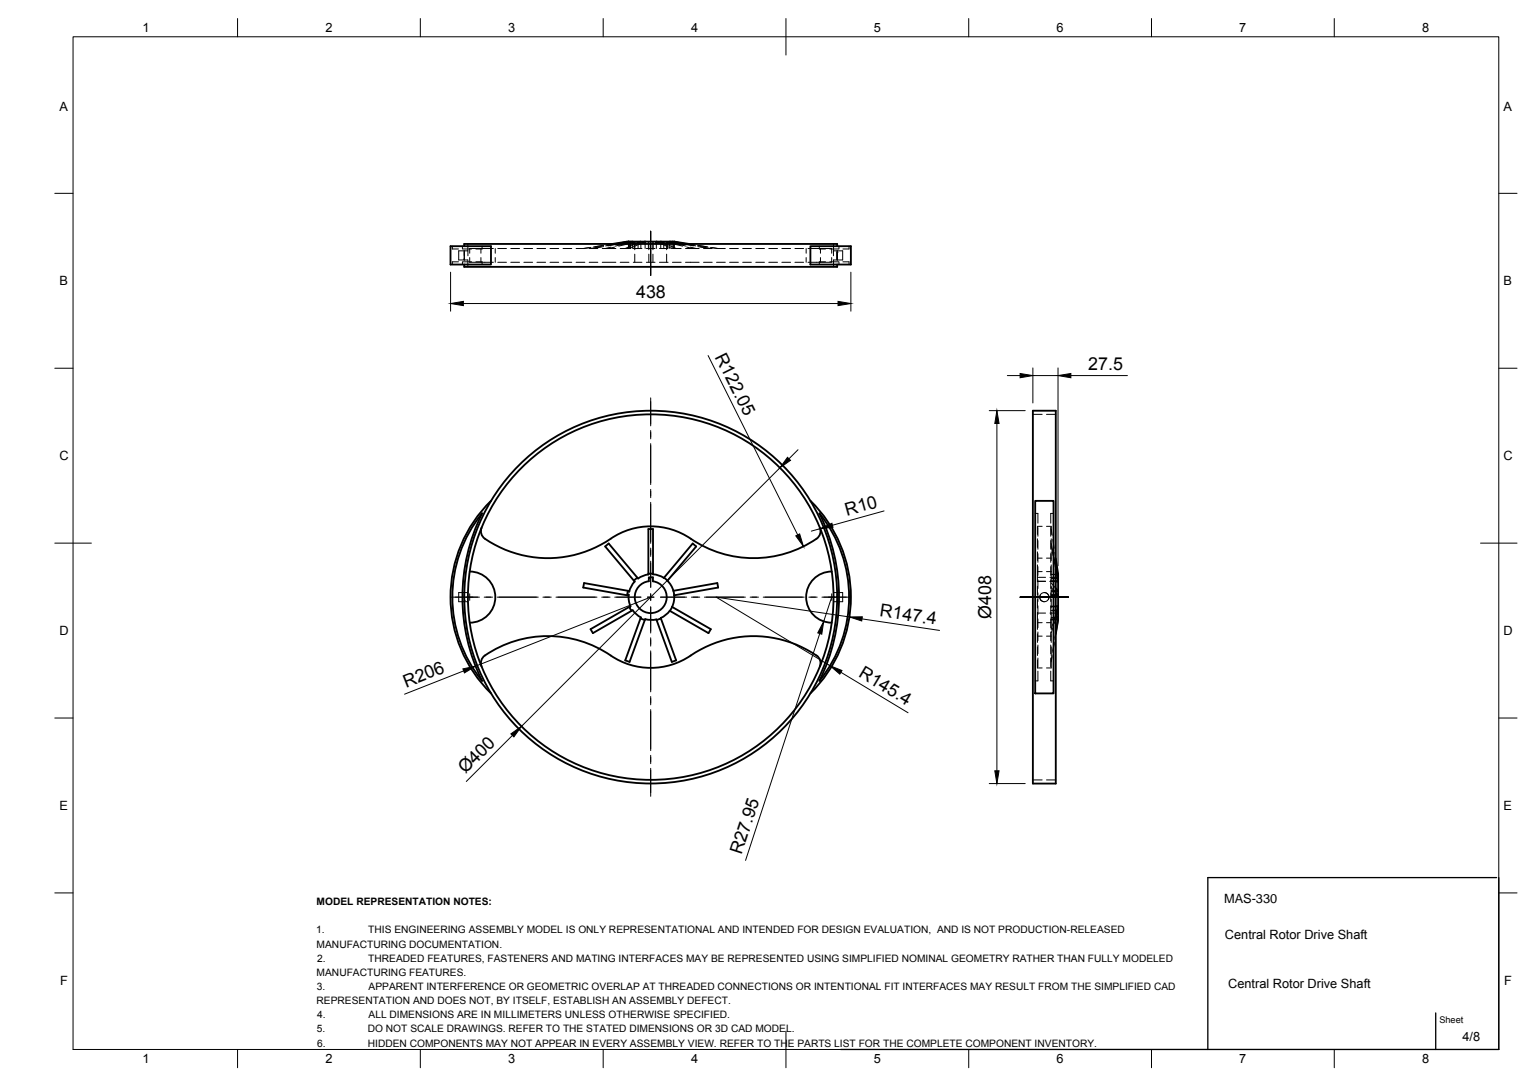
ISO-10303-21;
HEADER;
/* Generated by software containing ST-Developer
 * from STEP Tools, Inc. (www.steptools.com) 
 */

FILE_DESCRIPTION(
/* description */ ('STEP AP214'),
/* implementation_level */ '2;1');

FILE_NAME(
/* name */ 'Central Rotor Drive Shaft.step',
/* time_stamp */ '2026-10-12T14:05:15-07:00',
/* author */ (''),
/* organization */ (''),
/* preprocessor_version */ 'ST-DEVELOPER v20.2',
/* originating_system */ 'Autodesk Translation Framework v15.15.0.0',
/* authorisation */ '');

FILE_SCHEMA (('AUTOMOTIVE_DESIGN { 1 0 10303 214 3 1 1 }'));
ENDSEC;

DATA;
#10=MECHANICAL_DESIGN_GEOMETRIC_PRESENTATION_REPRESENTATION('',(#283),#39959);
#244=B_SPLINE_SURFACE_WITH_KNOTS('',3,1,((#26297,#26298),(#26299,#26300),
(#26301,#26302),(#26303,#26304),(#26305,#26306),(#26307,#26308),(#26309,
#26310),(#26311,#26312),(#26313,#26314),(#26315,#26316)),.UNSPECIFIED.,
 .F.,.F.,.F.,(4,2,2,2,4),(2,2),(0.5,0.625,0.75,0.875,1.),(0.,1.),
 .UNSPECIFIED.);
#245=B_SPLINE_SURFACE_WITH_KNOTS('',3,1,((#26363,#26364),(#26365,#26366),
(#26367,#26368),(#26369,#26370),(#26371,#26372),(#26373,#26374),(#26375,
#26376),(#26377,#26378),(#26379,#26380),(#26381,#26382),(#26383,#26384),
(#26385,#26386)),.UNSPECIFIED.,.F.,.F.,.F.,(4,2,2,2,2,4),(2,2),(0.,0.125,
0.25,0.375,0.5,0.503056895069501),(0.,1.),.UNSPECIFIED.);
#246=B_SPLINE_SURFACE_WITH_KNOTS('',3,1,((#27108,#27109),(#27110,#27111),
(#27112,#27113),(#27114,#27115),(#27116,#27117),(#27118,#27119),(#27120,
#27121),(#27122,#27123),(#27124,#27125),(#27126,#27127)),.UNSPECIFIED.,
 .F.,.F.,.F.,(4,2,2,2,4),(2,2),(0.5,0.625,0.75,0.875,1.00000000012908),
(0.,1.),.UNSPECIFIED.);
#247=B_SPLINE_SURFACE_WITH_KNOTS('',3,1,((#27130,#27131),(#27132,#27133),
(#27134,#27135),(#27136,#27137),(#27138,#27139),(#27140,#27141),(#27142,
#27143),(#27144,#27145),(#27146,#27147),(#27148,#27149),(#27150,#27151),
(#27152,#27153)),.UNSPECIFIED.,.F.,.F.,.F.,(4,2,2,2,2,4),(2,2),(0.,0.125,
0.25,0.375,0.5,0.50305689506972),(0.,1.),.UNSPECIFIED.);
#269=SHAPE_REPRESENTATION_RELATIONSHIP('SRR','None',#40003,#276);
#276=ADVANCED_BREP_SHAPE_REPRESENTATION('',(#291),#39953);
#283=STYLED_ITEM('',(#40046),#291);
#291=MANIFOLD_SOLID_BREP('Body1',#18260);
#341=PLANE('',#18548);
#342=PLANE('',#18550);
#343=PLANE('',#18554);
#344=PLANE('',#18559);
#345=PLANE('',#18560);
#346=PLANE('',#18580);
#347=PLANE('',#18583);
#348=PLANE('',#18588);
#349=PLANE('',#18593);
#350=PLANE('',#18594);
#351=PLANE('',#18632);
#352=PLANE('',#18666);
#353=PLANE('',#18667);
#354=PLANE('',#18680);
#355=PLANE('',#18684);
#356=PLANE('',#18686);
#357=PLANE('',#18687);
#358=PLANE('',#18688);
#359=PLANE('',#18689);
#360=PLANE('',#18690);
#361=PLANE('',#18691);
#362=PLANE('',#18692);
#363=PLANE('',#18693);
#364=PLANE('',#18694);
#365=PLANE('',#18695);
#366=PLANE('',#18696);
#367=PLANE('',#18697);
#368=PLANE('',#18698);
#369=PLANE('',#18699);
#370=PLANE('',#18700);
#371=PLANE('',#18701);
#372=PLANE('',#18702);
#373=PLANE('',#18703);
#374=PLANE('',#18704);
#375=PLANE('',#18705);
#376=PLANE('',#18706);
#377=PLANE('',#18707);
#378=PLANE('',#18708);
#379=PLANE('',#18709);
#380=PLANE('',#18710);
#381=PLANE('',#18711);
#382=PLANE('',#18712);
#383=PLANE('',#18713);
#384=PLANE('',#18714);
#385=PLANE('',#18715);
#386=PLANE('',#18718);
#387=PLANE('',#18719);
#388=PLANE('',#18720);
#935=FACE_BOUND('',#5965,.T.);
#936=FACE_BOUND('',#5967,.T.);
#937=FACE_BOUND('',#5986,.T.);
#938=FACE_BOUND('',#5988,.T.);
#939=FACE_BOUND('',#5994,.T.);
#940=FACE_BOUND('',#5995,.T.);
#941=FACE_BOUND('',#5997,.T.);
#942=FACE_BOUND('',#5998,.T.);
#943=FACE_BOUND('',#6010,.T.);
#944=FACE_BOUND('',#6012,.T.);
#945=FACE_BOUND('',#6013,.T.);
#946=FACE_BOUND('',#6014,.T.);
#947=FACE_BOUND('',#6015,.T.);
#948=FACE_BOUND('',#6016,.T.);
#949=FACE_BOUND('',#6018,.T.);
#950=FACE_BOUND('',#6028,.T.);
#951=FACE_BOUND('',#6030,.T.);
#952=FACE_BOUND('',#6038,.T.);
#953=FACE_BOUND('',#6040,.T.);
#1069=B_SPLINE_CURVE_WITH_KNOTS('',3,(#25647,#25648,#25649,#25650,#25651,
#25652),.UNSPECIFIED.,.F.,.F.,(4,2,4),(0.376702875081531,0.565054310328979,
0.753405745576428),.UNSPECIFIED.);
#1070=B_SPLINE_CURVE_WITH_KNOTS('',3,(#25654,#25655,#25656,#25657,#25658,
#25659),.UNSPECIFIED.,.F.,.F.,(4,2,4),(0.000204272915071079,0.188351437540765,
0.376680075941862),.UNSPECIFIED.);
#1071=B_SPLINE_CURVE_WITH_KNOTS('',3,(#25661,#25662,#25663,#25664,#25665,
#25666,#25667,#25668,#25669),.UNSPECIFIED.,.F.,.F.,(4,2,3,4),(2.63715317341441,
2.82527154476495,3.01362298230571,3.01382725522078),.UNSPECIFIED.);
#1072=B_SPLINE_CURVE_WITH_KNOTS('',3,(#25671,#25672,#25673,#25674,#25675,
#25676,#25677,#25678),.UNSPECIFIED.,.F.,.F.,(4,2,2,4),(2.26024327400092,
2.44856867197673,2.63692010722418,2.63715317341441),.UNSPECIFIED.);
#1073=B_SPLINE_CURVE_WITH_KNOTS('',3,(#25680,#25681,#25682,#25683,#25684,
#25685),.UNSPECIFIED.,.F.,.F.,(4,2,4),(1.88394027377768,2.07186580148184,
2.26021723672928),.UNSPECIFIED.);
#1074=B_SPLINE_CURVE_WITH_KNOTS('',3,(#25687,#25688,#25689,#25690,#25691,
#25692,#25693,#25694),.UNSPECIFIED.,.F.,.F.,(4,2,2,4),(1.5073284029247,
1.69516292869362,1.88351436623439,1.88394027377768),.UNSPECIFIED.);
#1075=B_SPLINE_CURVE_WITH_KNOTS('',3,(#25696,#25697,#25698,#25699,#25700,
#25701,#25702,#25703),.UNSPECIFIED.,.F.,.F.,(4,2,2,4),(1.13044830756701,
1.31846005361209,1.50681149115286,1.5073284029247),.UNSPECIFIED.);
#1076=B_SPLINE_CURVE_WITH_KNOTS('',3,(#25704,#25705,#25706,#25707,#25708,
#25709,#25710,#25711),.UNSPECIFIED.,.F.,.F.,(4,2,2,4),(0.753405745576428,
0.941757180823877,1.13010861607133,1.13044830756701),.UNSPECIFIED.);
#1077=B_SPLINE_CURVE_WITH_KNOTS('',3,(#25741,#25742,#25743,#25744,#25745,
#25746,#25747,#25748,#25749,#25750,#25751,#25752,#25753,#25754,#25755,#25756,
#25757,#25758,#25759,#25760,#25761,#25762,#25763,#25764,#25765,#25766,#25767,
#25768,#25769,#25770,#25771,#25772,#25773,#25774,#25775,#25776,#25777,#25778,
#25779,#25780,#25781,#25782,#25783,#25784,#25785,#25786,#25787,#25788,#25789,
#25790,#25791,#25792,#25793,#25794,#25795,#25796,#25797,#25798),
 .UNSPECIFIED.,.F.,.F.,(4,3,3,3,3,3,3,3,3,3,3,3,3,3,3,3,3,3,3,4),(0.124997637865204,
0.125004803698825,0.125015258789063,0.134771361364135,0.14467040638079,
0.154662369733195,0.164672368730329,0.174624579474319,0.184411644454489,
0.187522888183594,0.197283569985428,0.207159003809817,0.217118120942224,
0.21877670288086,0.227396265155205,0.2359533648241,0.244350344839939,0.250020612142817,
0.250030517578125,0.250040203921046),.UNSPECIFIED.);
#1078=B_SPLINE_CURVE_WITH_KNOTS('',3,(#25800,#25801,#25802,#25803,#25804,
#25805,#25806,#25807,#25808,#25809,#25810,#25811,#25812,#25813,#25814,#25815,
#25816,#25817,#25818,#25819,#25820,#25821,#25822,#25823,#25824,#25825,#25826,
#25827,#25828,#25829,#25830,#25831,#25832,#25833,#25834,#25835,#25836),
 .UNSPECIFIED.,.F.,.F.,(4,3,3,3,3,3,3,3,3,3,3,3,4),(0.,0.0100788585654741,
0.0205391817562645,0.0308655410000762,0.04118079735384,0.0514218014928902,
0.0620067121426169,0.0630819969569995,0.0730857845910175,0.0834236143414073,
0.093761444091797,0.118957117023634,0.124997637865204),.UNSPECIFIED.);
#1079=B_SPLINE_CURVE_WITH_KNOTS('',3,(#25838,#25839,#25840,#25841,#25842,
#25843,#25844,#25845,#25846,#25847,#25848,#25849,#25850,#25851,#25852,#25853,
#25854,#25855,#25856,#25857,#25858,#25859,#25860,#25861,#25862,#25863,#25864,
#25865,#25866,#25867,#25868,#25869,#25870,#25871,#25872,#25873,#25874,#25875,
#25876,#25877,#25878,#25879,#25880,#25881,#25882,#25883,#25884,#25885,#25886,
#25887,#25888,#25889),.UNSPECIFIED.,.F.,.F.,(4,3,3,3,3,3,3,3,3,3,3,3,3,
3,3,3,3,4),(0.875010334230379,0.875015258789063,0.885063223983587,0.895662334037692,
0.906261444091797,0.915329176293059,0.924362963681523,0.933304455697802,
0.935941078938443,0.937102710968539,0.938038619544317,0.948083027116603,
0.95824477230157,0.968683579226177,0.978878572825813,0.989439286412907,
0.999400899492149,1.),.UNSPECIFIED.);
#1080=B_SPLINE_CURVE_WITH_KNOTS('',3,(#25891,#25892,#25893,#25894,#25895,
#25896,#25897,#25898,#25899,#25900,#25901,#25902,#25903,#25904,#25905,#25906,
#25907,#25908,#25909,#25910,#25911,#25912,#25913,#25914,#25915,#25916,#25917,
#25918,#25919,#25920,#25921,#25922,#25923,#25924,#25925,#25926,#25927,#25928,
#25929,#25930,#25931,#25932,#25933,#25934,#25935,#25936,#25937,#25938,#25939,
#25940,#25941,#25942),.UNSPECIFIED.,.F.,.F.,(4,3,3,3,3,3,3,3,3,3,3,3,3,
3,3,3,3,4),(0.750027510254452,0.750030180562894,0.750030517578125,0.760114469760994,
0.770326204646331,0.780875375530647,0.791169951965582,0.801846420074588,
0.811924599407989,0.812522888183594,0.822590381964961,0.832779920362826,
0.84333280346223,0.853563394247635,0.863720399981247,0.873715992551155,
0.874991452760439,0.875010334230379),.UNSPECIFIED.);
#1081=B_SPLINE_CURVE_WITH_KNOTS('',3,(#25944,#25945,#25946,#25947,#25948,
#25949,#25950,#25951,#25952,#25953,#25954,#25955,#25956,#25957,#25958,#25959,
#25960,#25961,#25962,#25963,#25964,#25965,#25966,#25967,#25968,#25969,#25970,
#25971,#25972,#25973,#25974,#25975,#25976,#25977,#25978,#25979,#25980,#25981,
#25982,#25983,#25984,#25985,#25986,#25987,#25988,#25989),.UNSPECIFIED.,
 .F.,.F.,(4,3,3,3,3,3,3,3,3,3,3,3,3,3,3,4),(0.625035680662314,0.625045776367188,
0.634959360244037,0.645005190259783,0.655638429438002,0.66577810723537,
0.675860402489048,0.685791959316116,0.687538146972657,0.697444002791749,
0.707465979715092,0.71754735415445,0.727602770201362,0.737586421487148,
0.747408036910529,0.750027510254452),.UNSPECIFIED.);
#1082=B_SPLINE_CURVE_WITH_KNOTS('',3,(#25991,#25992,#25993,#25994,#25995,
#25996,#25997,#25998,#25999,#26000,#26001,#26002,#26003,#26004,#26005,#26006,
#26007,#26008,#26009,#26010,#26011,#26012,#26013,#26014,#26015,#26016,#26017,
#26018,#26019,#26020,#26021,#26022,#26023,#26024,#26025,#26026,#26027,#26028,
#26029,#26030,#26031,#26032,#26033,#26034,#26035,#26036,#26037,#26038,#26039,
#26040,#26041,#26042,#26043,#26044,#26045),.UNSPECIFIED.,.F.,.F.,(4,3,3,
3,3,3,3,3,3,3,3,3,3,3,3,3,3,3,4),(0.500061035156251,0.509784082219549,0.519668083969381,
0.529684204027609,0.539699455781287,0.549643684996335,0.559453770503833,
0.561600384288871,0.562427817012746,0.563166095090099,0.572935702006583,
0.582817729960924,0.592779134388661,0.593799591064454,0.602508339696414,
0.611153433496651,0.619637704379647,0.625016883677845,0.625035680662314),
 .UNSPECIFIED.);
#1083=B_SPLINE_CURVE_WITH_KNOTS('',3,(#26047,#26048,#26049,#26050,#26051,
#26052,#26053,#26054,#26055,#26056,#26057,#26058,#26059,#26060,#26061,#26062,
#26063,#26064,#26065,#26066,#26067,#26068,#26069,#26070,#26071,#26072,#26073,
#26074,#26075,#26076,#26077,#26078,#26079,#26080,#26081,#26082,#26083,#26084,
#26085,#26086,#26087,#26088,#26089,#26090,#26091,#26092),.UNSPECIFIED.,
 .F.,.F.,(4,3,3,3,3,3,3,3,3,3,3,3,3,3,3,4),(0.375039662445796,0.375045776367188,
0.385157469228026,0.395395289459459,0.405934818535024,0.416252083475239,
0.426902744618479,0.437004013717147,0.437553405761719,0.447532078985895,
0.45761507319284,0.4677726888567,0.468807220458985,0.491821180845468,0.500004452744443,
0.500032744006821),.UNSPECIFIED.);
#1084=B_SPLINE_CURVE_WITH_KNOTS('',3,(#26094,#26095,#26096,#26097,#26098,
#26099,#26100,#26101,#26102,#26103,#26104,#26105,#26106,#26107,#26108,#26109,
#26110,#26111,#26112,#26113,#26114,#26115,#26116,#26117,#26118,#26119,#26120,
#26121,#26122,#26123,#26124,#26125,#26126,#26127,#26128,#26129,#26130,#26131,
#26132,#26133,#26134,#26135,#26136,#26137,#26138,#26139),.UNSPECIFIED.,
 .F.,.F.,(4,3,3,3,3,3,3,3,3,3,3,3,3,3,3,4),(0.250040203921046,0.260006897061865,
0.270104787324373,0.280713127236444,0.290902669953587,0.301034854339568,
0.311017727734801,0.312538146972657,0.322520836674231,0.332620319240001,
0.34322347142839,0.353356467748657,0.363416849810154,0.373318487372145,
0.375032927993557,0.375039662445796),.UNSPECIFIED.);
#1085=B_SPLINE_CURVE_WITH_KNOTS('',3,(#26158,#26159,#26160,#26161,#26162,
#26163,#26164,#26165),.UNSPECIFIED.,.F.,.F.,(4,2,2,4),(1.88326006932265,
1.88351436623439,2.07186580148184,2.2601469129838),.UNSPECIFIED.);
#1086=B_SPLINE_CURVE_WITH_KNOTS('',3,(#26167,#26168,#26169,#26170,#26171,
#26172,#26173,#26174),.UNSPECIFIED.,.F.,.F.,(4,2,2,4),(1.50654556057706,
1.50681149115286,1.69516292869362,1.88326006932265),.UNSPECIFIED.);
#1087=B_SPLINE_CURVE_WITH_KNOTS('',3,(#26176,#26177,#26178,#26179,#26180,
#26181),.UNSPECIFIED.,.F.,.F.,(4,2,4),(1.13015385044563,1.31846005361209,
1.50654556057706),.UNSPECIFIED.);
#1088=B_SPLINE_CURVE_WITH_KNOTS('',3,(#26183,#26184,#26185,#26186,#26187,
#26188),.UNSPECIFIED.,.F.,.F.,(4,2,4),(0.753405745576428,0.941757180823877,
1.13010861607133),.UNSPECIFIED.);
#1089=B_SPLINE_CURVE_WITH_KNOTS('',3,(#26190,#26191,#26192,#26193,#26194,
#26195,#26196,#26197),.UNSPECIFIED.,.F.,.F.,(4,2,2,4),(0.376303807212213,
0.376702875081531,0.565054310328979,0.753405745576428),.UNSPECIFIED.);
#1090=B_SPLINE_CURVE_WITH_KNOTS('',3,(#26199,#26200,#26201,#26202,#26203,
#26204,#26205,#26206,#26207),.UNSPECIFIED.,.F.,.F.,(4,3,2,4),(3.01311448574183,
3.01362298230571,3.20197441984648,3.38992678951793),.UNSPECIFIED.);
#1091=B_SPLINE_CURVE_WITH_KNOTS('',3,(#26209,#26210,#26211,#26212,#26213,
#26214,#26215,#26216),.UNSPECIFIED.,.F.,.F.,(4,2,2,4),(2.63643507955563,
2.63692010722418,2.82527154476495,3.01311448574183),.UNSPECIFIED.);
#1092=B_SPLINE_CURVE_WITH_KNOTS('',3,(#26217,#26218,#26219,#26220,#26221,
#26222),.UNSPECIFIED.,.F.,.F.,(4,2,4),(2.26021723672928,2.44856867197673,
2.63643507955563),.UNSPECIFIED.);
#1093=B_SPLINE_CURVE_WITH_KNOTS('',3,(#26256,#26257,#26258,#26259),
 .UNSPECIFIED.,.F.,.F.,(4,4),(0.874999999999996,1.),.UNSPECIFIED.);
#1094=B_SPLINE_CURVE_WITH_KNOTS('',3,(#26261,#26262,#26263,#26264),
 .UNSPECIFIED.,.F.,.F.,(4,4),(0.,0.124999999999996),.UNSPECIFIED.);
#1095=B_SPLINE_CURVE_WITH_KNOTS('',3,(#26266,#26267,#26268,#26269),
 .UNSPECIFIED.,.F.,.F.,(4,4),(0.124999999999996,0.249999999999992),
 .UNSPECIFIED.);
#1096=B_SPLINE_CURVE_WITH_KNOTS('',3,(#26271,#26272,#26273,#26274),
 .UNSPECIFIED.,.F.,.F.,(4,4),(0.249999999999992,0.374999999999988),
 .UNSPECIFIED.);
#1097=B_SPLINE_CURVE_WITH_KNOTS('',3,(#26276,#26277,#26278,#26279,#26280,
#26281),.UNSPECIFIED.,.F.,.F.,(4,2,4),(0.375000000250893,0.499999999999984,
0.500028277877377),.UNSPECIFIED.);
#1098=B_SPLINE_CURVE_WITH_KNOTS('',3,(#26283,#26284,#26285,#26286),
 .UNSPECIFIED.,.F.,.F.,(4,4),(0.50005655573509,0.624999999999988),
 .UNSPECIFIED.);
#1099=B_SPLINE_CURVE_WITH_KNOTS('',3,(#26288,#26289,#26290,#26291),
 .UNSPECIFIED.,.F.,.F.,(4,4),(0.624999999999988,0.749999999999992),
 .UNSPECIFIED.);
#1100=B_SPLINE_CURVE_WITH_KNOTS('',3,(#26293,#26294,#26295,#26296),
 .UNSPECIFIED.,.F.,.F.,(4,4),(0.749999999999992,0.874999999999996),
 .UNSPECIFIED.);
#1101=B_SPLINE_CURVE_WITH_KNOTS('',3,(#26320,#26321,#26322,#26323,#26324,
#26325,#26326,#26327,#26328,#26329,#26330,#26331,#26332,#26333,#26334,#26335,
#26336,#26337,#26338,#26339,#26340,#26341,#26342,#26343),.UNSPECIFIED.,
 .F.,.F.,(4,2,2,2,2,2,2,2,2,2,2,4),(0.,0.103381366704768,0.206922202201336,
0.391377450354442,0.488690558489562,0.58707753918209,0.772543406462477,
0.970634500277933,1.19532551051909,1.24886321535489,1.45372318457095,1.6598018219901),
 .UNSPECIFIED.);
#1102=B_SPLINE_CURVE_WITH_KNOTS('',3,(#26390,#26391,#26392,#26393,#26394,
#26395,#26396,#26397,#26398,#26399,#26400,#26401,#26402,#26403,#26404,#26405,
#26406,#26407,#26408,#26409,#26410,#26411,#26412,#26413,#26414,#26415,#26416,
#26417,#26418,#26419,#26420,#26421,#26422,#26423,#26424,#26425,#26426,#26427,
#26428,#26429,#26430,#26431,#26432,#26433,#26434,#26435,#26436,#26437,#26438,
#26439,#26440,#26441,#26442,#26443,#26444,#26445,#26446,#26447,#26448,#26449,
#26450,#26451,#26452,#26453,#26454,#26455,#26456,#26457,#26458,#26459,#26460,
#26461,#26462,#26463,#26464,#26465,#26466,#26467,#26468,#26469,#26470,#26471,
#26472,#26473,#26474,#26475,#26476,#26477,#26478,#26479,#26480,#26481,#26482,
#26483,#26484,#26485,#26486,#26487,#26488,#26489,#26490,#26491,#26492,#26493,
#26494,#26495,#26496,#26497,#26498,#26499,#26500,#26501,#26502,#26503,#26504,
#26505,#26506,#26507,#26508,#26509,#26510,#26511,#26512,#26513,#26514,#26515,
#26516,#26517,#26518,#26519,#26520,#26521,#26522,#26523,#26524,#26525,#26526,
#26527,#26528,#26529,#26530,#26531,#26532,#26533,#26534,#26535,#26536,#26537,
#26538,#26539,#26540,#26541,#26542,#26543,#26544,#26545,#26546,#26547,#26548,
#26549,#26550,#26551,#26552,#26553,#26554,#26555,#26556,#26557,#26558,#26559,
#26560,#26561),.UNSPECIFIED.,.F.,.F.,(4,3,3,3,3,3,3,3,3,3,3,3,3,3,3,3,3,
3,3,3,3,3,3,3,3,3,3,3,3,3,3,3,3,3,3,3,3,3,3,3,3,3,3,3,3,3,3,3,3,3,3,3,3,
3,3,3,3,4),(0.,0.000315375744567924,0.000645903817980758,0.000976431891393592,
0.0012812537484511,0.00158740068641533,0.00189480456358316,0.00195286378278718,
0.00227229401054678,0.00260079484236378,0.00292929567418078,0.00320274758832941,
0.00347469402173951,0.00374433547800945,0.00390572756557437,0.00390584133492772,
0.00421689206020479,0.00453088806273884,0.00484662827091633,0.00488215945696796,
0.00525366301006075,0.00562563969088054,0.00585859134836155,0.00638053264119389,
0.00683502323975515,0.00715062223032276,0.00748103868073575,0.00779159828439098,
0.00781145513114874,0.00781203150209657,0.00808972377000141,0.00836905928236821,
0.00865075449187036,0.00878788702254233,0.00910517886612052,0.00943474889002822,
0.00976431891393592,0.0100622297668594,0.0103592836570688,0.0106546119602171,
0.0107407508053295,0.0110626953843491,0.0113899390405361,0.0117171826967231,
0.0117180975894192,0.0121313722590175,0.0125539529147115,0.0126936145881167,
0.0130183666566513,0.0133457392744377,0.0136700464795103,0.0139888224703152,
0.0143176504206095,0.0146464783709039,0.014919070754581,0.015190101683422,
0.0154587424133886,0.0156229102622975),.UNSPECIFIED.);
#1103=B_SPLINE_CURVE_WITH_KNOTS('',3,(#26602,#26603,#26604,#26605),
 .UNSPECIFIED.,.F.,.F.,(4,4),(-0.00017716250113245,0.),.UNSPECIFIED.);
#1104=B_SPLINE_CURVE_WITH_KNOTS('',3,(#26609,#26610,#26611,#26612,#26613,
#26614,#26615,#26616,#26617,#26618,#26619,#26620,#26621,#26622,#26623,#26624,
#26625,#26626,#26627,#26628,#26629,#26630,#26631,#26632),.UNSPECIFIED.,
 .F.,.F.,(4,2,2,2,2,2,2,2,2,2,2,4),(-1.65980182253606,-1.45372318489466,
-1.24886321541509,-1.19532551060548,-0.970634500303615,-0.772543406460149,
-0.587077539177558,-0.488690558484114,-0.391377450348774,-0.20692220219487,
-0.103381366701537,-0.00017716250113245),.UNSPECIFIED.);
#1105=B_SPLINE_CURVE_WITH_KNOTS('',3,(#26633,#26634,#26635,#26636,#26637,
#26638,#26639,#26640,#26641,#26642,#26643,#26644,#26645,#26646,#26647,#26648,
#26649,#26650,#26651,#26652,#26653,#26654,#26655,#26656,#26657,#26658,#26659,
#26660,#26661,#26662,#26663,#26664,#26665,#26666,#26667,#26668,#26669,#26670,
#26671,#26672,#26673,#26674,#26675,#26676,#26677,#26678,#26679,#26680,#26681,
#26682,#26683,#26684,#26685,#26686,#26687,#26688,#26689,#26690,#26691,#26692,
#26693,#26694,#26695,#26696,#26697,#26698,#26699,#26700,#26701,#26702,#26703,
#26704,#26705,#26706,#26707,#26708,#26709,#26710,#26711,#26712,#26713,#26714,
#26715,#26716,#26717,#26718,#26719,#26720,#26721,#26722,#26723,#26724,#26725,
#26726,#26727,#26728,#26729,#26730,#26731,#26732,#26733,#26734,#26735,#26736,
#26737,#26738,#26739,#26740,#26741,#26742,#26743,#26744,#26745,#26746,#26747,
#26748,#26749,#26750,#26751,#26752,#26753,#26754,#26755,#26756,#26757,#26758,
#26759,#26760,#26761,#26762,#26763,#26764,#26765,#26766,#26767,#26768,#26769,
#26770,#26771,#26772,#26773,#26774,#26775,#26776,#26777,#26778,#26779,#26780,
#26781,#26782,#26783,#26784,#26785,#26786,#26787,#26788,#26789,#26790,#26791,
#26792,#26793,#26794,#26795,#26796,#26797,#26798,#26799,#26800,#26801,#26802,
#26803,#26804),.UNSPECIFIED.,.F.,.F.,(4,3,3,3,3,3,3,3,3,3,3,3,3,3,3,3,3,
3,3,3,3,3,3,3,3,3,3,3,3,3,3,3,3,3,3,3,3,3,3,3,3,3,3,3,3,3,3,3,3,3,3,3,3,
3,3,3,3,4),(4.21060351010033E-19,0.000315375742575029,0.000645903817003116,
0.000976431891431204,0.00128125374781883,0.00158740068510089,0.0018948045615801,
0.00195286378286241,0.00227229401064095,0.00260079484246728,0.00292929567429361,
0.00320274758882887,0.00347469402262506,0.00374433547927827,0.00390572756572481,
0.00390584133502637,0.00421689206038293,0.00453088806297221,0.00484662827116357,
0.00488215945715601,0.00525366301724405,0.00562563970480409,0.00585859134858722,
0.00638053260631128,0.00683502324001842,0.00715062223061402,0.00748103868103182,
0.0077915982846478,0.00781145513144962,0.00781203150237952,0.00808972376946302,
0.00836905928099522,0.00865075448965919,0.00878788702288083,0.00910517886651736,
0.0094347488904147,0.00976431891431203,0.0100622297685835,0.01035928366013,
0.0106546119645884,0.0107407508057432,0.0110626953846664,0.0113899390409204,
0.0117171826971744,0.0117180975897762,0.01213137223928,0.0125539528739886,
0.0126936145886056,0.0130183666541618,0.0133457392688836,0.0136700464800368,
0.0139888224708903,0.0143176504211792,0.014646478371468,0.0149190707552556,
0.015190101684208,0.0154587424142883,0.0156229102628992),.UNSPECIFIED.);
#1535=LINE('',#25634,#3108);
#1536=LINE('',#25637,#3109);
#1537=LINE('',#25645,#3110);
#1538=LINE('',#25717,#3111);
#1539=LINE('',#25720,#3112);
#1540=LINE('',#25732,#3113);
#1541=LINE('',#25735,#3114);
#1542=LINE('',#26145,#3115);
#1543=LINE('',#26148,#3116);
#1544=LINE('',#26156,#3117);
#1545=LINE('',#26228,#3118);
#1546=LINE('',#26231,#3119);
#1547=LINE('',#26247,#3120);
#1548=LINE('',#26250,#3121);
#1549=LINE('',#26318,#3122);
#1550=LINE('',#26344,#3123);
#1551=LINE('',#26350,#3124);
#1552=LINE('',#26353,#3125);
#1553=LINE('',#26359,#3126);
#1554=LINE('',#26362,#3127);
#1555=LINE('',#26388,#3128);
#1556=LINE('',#26562,#3129);
#1557=LINE('',#26568,#3130);
#1558=LINE('',#26571,#3131);
#1559=LINE('',#26577,#3132);
#1560=LINE('',#26580,#3133);
#1561=LINE('',#26586,#3134);
#1562=LINE('',#26589,#3135);
#1563=LINE('',#26593,#3136);
#1564=LINE('',#26595,#3137);
#1565=LINE('',#26600,#3138);
#1566=LINE('',#26607,#3139);
#1567=LINE('',#26809,#3140);
#1568=LINE('',#26812,#3141);
#1569=LINE('',#26818,#3142);
#1570=LINE('',#26823,#3143);
#1571=LINE('',#26843,#3144);
#1572=LINE('',#26845,#3145);
#1573=LINE('',#26849,#3146);
#1574=LINE('',#26851,#3147);
#1575=LINE('',#26852,#3148);
#1576=LINE('',#26854,#3149);
#1577=LINE('',#26856,#3150);
#1578=LINE('',#26858,#3151);
#1579=LINE('',#26862,#3152);
#1580=LINE('',#26864,#3153);
#1581=LINE('',#26866,#3154);
#1582=LINE('',#26870,#3155);
#1583=LINE('',#26872,#3156);
#1584=LINE('',#26874,#3157);
#1585=LINE('',#26878,#3158);
#1586=LINE('',#26880,#3159);
#1587=LINE('',#26882,#3160);
#1588=LINE('',#26884,#3161);
#1589=LINE('',#26888,#3162);
#1590=LINE('',#26890,#3163);
#1591=LINE('',#26892,#3164);
#1592=LINE('',#26894,#3165);
#1593=LINE('',#26896,#3166);
#1594=LINE('',#26900,#3167);
#1595=LINE('',#26902,#3168);
#1596=LINE('',#26904,#3169);
#1597=LINE('',#26908,#3170);
#1598=LINE('',#26910,#3171);
#1599=LINE('',#26912,#3172);
#1600=LINE('',#26915,#3173);
#1601=LINE('',#26918,#3174);
#1602=LINE('',#26921,#3175);
#1603=LINE('',#26924,#3176);
#1604=LINE('',#26927,#3177);
#1605=LINE('',#26930,#3178);
#1606=LINE('',#26933,#3179);
#1607=LINE('',#26936,#3180);
#1608=LINE('',#26939,#3181);
#1609=LINE('',#26942,#3182);
#1610=LINE('',#26945,#3183);
#1611=LINE('',#26948,#3184);
#1612=LINE('',#26950,#3185);
#1613=LINE('',#26954,#3186);
#1614=LINE('',#26957,#3187);
#1615=LINE('',#26960,#3188);
#1616=LINE('',#26963,#3189);
#1617=LINE('',#26968,#3190);
#1618=LINE('',#26971,#3191);
#1619=LINE('',#26975,#3192);
#1620=LINE('',#26981,#3193);
#1621=LINE('',#26985,#3194);
#1622=LINE('',#26989,#3195);
#1623=LINE('',#26995,#3196);
#1624=LINE('',#26997,#3197);
#1625=LINE('',#26998,#3198);
#1626=LINE('',#27001,#3199);
#1627=LINE('',#27003,#3200);
#1628=LINE('',#27004,#3201);
#1629=LINE('',#27006,#3202);
#1630=LINE('',#27008,#3203);
#1631=LINE('',#27009,#3204);
#1632=LINE('',#27011,#3205);
#1633=LINE('',#27013,#3206);
#1634=LINE('',#27014,#3207);
#1635=LINE('',#27016,#3208);
#1636=LINE('',#27018,#3209);
#1637=LINE('',#27020,#3210);
#1638=LINE('',#27022,#3211);
#1639=LINE('',#27023,#3212);
#1640=LINE('',#27025,#3213);
#1641=LINE('',#27027,#3214);
#1642=LINE('',#27029,#3215);
#1643=LINE('',#27030,#3216);
#1644=LINE('',#27032,#3217);
#1645=LINE('',#27034,#3218);
#1646=LINE('',#27035,#3219);
#1647=LINE('',#27037,#3220);
#1648=LINE('',#27039,#3221);
#1649=LINE('',#27040,#3222);
#1650=LINE('',#27042,#3223);
#1651=LINE('',#27044,#3224);
#1652=LINE('',#27045,#3225);
#1653=LINE('',#27047,#3226);
#1654=LINE('',#27049,#3227);
#1655=LINE('',#27050,#3228);
#1656=LINE('',#27052,#3229);
#1657=LINE('',#27054,#3230);
#1658=LINE('',#27055,#3231);
#1659=LINE('',#27058,#3232);
#1660=LINE('',#27059,#3233);
#1661=LINE('',#27063,#3234);
#1662=LINE('',#27064,#3235);
#1663=LINE('',#27068,#3236);
#1664=LINE('',#27070,#3237);
#1665=LINE('',#27072,#3238);
#1666=LINE('',#27073,#3239);
#1667=LINE('',#27077,#3240);
#1668=LINE('',#27079,#3241);
#1669=LINE('',#27080,#3242);
#1670=LINE('',#27084,#3243);
#1671=LINE('',#27085,#3244);
#1672=LINE('',#27089,#3245);
#1673=LINE('',#27090,#3246);
#1674=LINE('',#27094,#3247);
#1675=LINE('',#27095,#3248);
#1676=LINE('',#27099,#3249);
#1677=LINE('',#27100,#3250);
#1678=LINE('',#27104,#3251);
#1679=LINE('',#27105,#3252);
#1680=LINE('',#27155,#3253);
#1681=LINE('',#27157,#3254);
#3108=VECTOR('',#20517,1000.);
#3109=VECTOR('',#20520,1000.);
#3110=VECTOR('',#20531,5.);
#3111=VECTOR('',#20536,10.);
#3112=VECTOR('',#20539,10.);
#3113=VECTOR('',#20556,1000.);
#3114=VECTOR('',#20559,1000.);
#3115=VECTOR('',#20588,1000.);
#3116=VECTOR('',#20591,1000.);
#3117=VECTOR('',#20602,5.);
#3118=VECTOR('',#20607,10.);
#3119=VECTOR('',#20610,10.);
#3120=VECTOR('',#20631,1000.);
#3121=VECTOR('',#20634,1000.);
#3122=VECTOR('',#20659,1000.);
#3123=VECTOR('',#20660,1000.);
#3124=VECTOR('',#20665,1000.);
#3125=VECTOR('',#20668,1000.);
#3126=VECTOR('',#20673,1000.);
#3127=VECTOR('',#20676,1000.);
#3128=VECTOR('',#20677,1000.);
#3129=VECTOR('',#20678,1000.);
#3130=VECTOR('',#20683,1000.);
#3131=VECTOR('',#20686,1000.);
#3132=VECTOR('',#20691,1000.);
#3133=VECTOR('',#20694,1000.);
#3134=VECTOR('',#20699,1000.);
#3135=VECTOR('',#20702,1000.);
#3136=VECTOR('',#20707,204.);
#3137=VECTOR('',#20708,204.);
#3138=VECTOR('',#20715,200.);
#3139=VECTOR('',#20716,200.);
#3140=VECTOR('',#20723,1000.);
#3141=VECTOR('',#20724,1000.);
#3142=VECTOR('',#20731,1000.);
#3143=VECTOR('',#20736,1000.);
#3144=VECTOR('',#20759,1000.);
#3145=VECTOR('',#20760,1000.);
#3146=VECTOR('',#20763,1000.);
#3147=VECTOR('',#20764,1000.);
#3148=VECTOR('',#20765,1000.);
#3149=VECTOR('',#20766,1000.);
#3150=VECTOR('',#20767,1000.);
#3151=VECTOR('',#20768,1000.);
#3152=VECTOR('',#20771,1000.);
#3153=VECTOR('',#20772,1000.);
#3154=VECTOR('',#20773,1000.);
#3155=VECTOR('',#20776,1000.);
#3156=VECTOR('',#20777,1000.);
#3157=VECTOR('',#20778,1000.);
#3158=VECTOR('',#20781,1000.);
#3159=VECTOR('',#20782,1000.);
#3160=VECTOR('',#20783,1000.);
#3161=VECTOR('',#20784,1000.);
#3162=VECTOR('',#20787,1000.);
#3163=VECTOR('',#20788,1000.);
#3164=VECTOR('',#20789,1000.);
#3165=VECTOR('',#20790,1000.);
#3166=VECTOR('',#20791,1000.);
#3167=VECTOR('',#20794,1000.);
#3168=VECTOR('',#20795,1000.);
#3169=VECTOR('',#20796,1000.);
#3170=VECTOR('',#20799,1000.);
#3171=VECTOR('',#20800,1000.);
#3172=VECTOR('',#20801,1000.);
#3173=VECTOR('',#20804,1000.);
#3174=VECTOR('',#20807,1000.);
#3175=VECTOR('',#20810,1000.);
#3176=VECTOR('',#20813,1000.);
#3177=VECTOR('',#20816,1000.);
#3178=VECTOR('',#20819,1000.);
#3179=VECTOR('',#20822,1000.);
#3180=VECTOR('',#20825,1000.);
#3181=VECTOR('',#20828,1000.);
#3182=VECTOR('',#20831,1000.);
#3183=VECTOR('',#20834,1000.);
#3184=VECTOR('',#20837,1000.);
#3185=VECTOR('',#20838,1000.);
#3186=VECTOR('',#20843,1000.);
#3187=VECTOR('',#20846,1000.);
#3188=VECTOR('',#20849,1000.);
#3189=VECTOR('',#20852,1000.);
#3190=VECTOR('',#20859,1000.);
#3191=VECTOR('',#20862,1000.);
#3192=VECTOR('',#20867,1000.);
#3193=VECTOR('',#20876,1000.);
#3194=VECTOR('',#20881,1000.);
#3195=VECTOR('',#20886,1000.);
#3196=VECTOR('',#20895,1000.);
#3197=VECTOR('',#20896,1000.);
#3198=VECTOR('',#20897,1000.);
#3199=VECTOR('',#20900,1000.);
#3200=VECTOR('',#20901,1000.);
#3201=VECTOR('',#20902,1000.);
#3202=VECTOR('',#20903,1000.);
#3203=VECTOR('',#20904,1000.);
#3204=VECTOR('',#20905,1000.);
#3205=VECTOR('',#20906,1000.);
#3206=VECTOR('',#20907,1000.);
#3207=VECTOR('',#20908,1000.);
#3208=VECTOR('',#20909,1000.);
#3209=VECTOR('',#20910,1000.);
#3210=VECTOR('',#20911,1000.);
#3211=VECTOR('',#20912,1000.);
#3212=VECTOR('',#20913,1000.);
#3213=VECTOR('',#20914,1000.);
#3214=VECTOR('',#20915,1000.);
#3215=VECTOR('',#20916,1000.);
#3216=VECTOR('',#20917,1000.);
#3217=VECTOR('',#20918,1000.);
#3218=VECTOR('',#20919,1000.);
#3219=VECTOR('',#20920,1000.);
#3220=VECTOR('',#20921,1000.);
#3221=VECTOR('',#20922,1000.);
#3222=VECTOR('',#20923,1000.);
#3223=VECTOR('',#20924,1000.);
#3224=VECTOR('',#20925,1000.);
#3225=VECTOR('',#20926,1000.);
#3226=VECTOR('',#20927,1000.);
#3227=VECTOR('',#20928,1000.);
#3228=VECTOR('',#20929,1000.);
#3229=VECTOR('',#20930,1000.);
#3230=VECTOR('',#20931,1000.);
#3231=VECTOR('',#20932,1000.);
#3232=VECTOR('',#20937,1000.);
#3233=VECTOR('',#20938,1000.);
#3234=VECTOR('',#20945,1000.);
#3235=VECTOR('',#20946,1000.);
#3236=VECTOR('',#20953,1000.);
#3237=VECTOR('',#20956,1000.);
#3238=VECTOR('',#20959,1000.);
#3239=VECTOR('',#20960,1000.);
#3240=VECTOR('',#20967,1000.);
#3241=VECTOR('',#20970,1000.);
#3242=VECTOR('',#20971,1000.);
#3243=VECTOR('',#20978,1000.);
#3244=VECTOR('',#20979,1000.);
#3245=VECTOR('',#20986,1000.);
#3246=VECTOR('',#20987,1000.);
#3247=VECTOR('',#20994,1000.);
#3248=VECTOR('',#20995,1000.);
#3249=VECTOR('',#21002,1000.);
#3250=VECTOR('',#21003,1000.);
#3251=VECTOR('',#21010,1000.);
#3252=VECTOR('',#21011,1000.);
#3253=VECTOR('',#21022,1000.);
#3254=VECTOR('',#21025,1000.);
#4594=CYLINDRICAL_SURFACE('',#18537,206.);
#4595=CYLINDRICAL_SURFACE('',#18540,145.404667636179);
#4596=CYLINDRICAL_SURFACE('',#18543,5.);
#4597=CYLINDRICAL_SURFACE('',#18545,147.404667636179);
#4598=CYLINDRICAL_SURFACE('',#18555,145.404667636179);
#4599=CYLINDRICAL_SURFACE('',#18557,206.);
#4600=CYLINDRICAL_SURFACE('',#18561,204.);
#4601=CYLINDRICAL_SURFACE('',#18562,204.);
#4602=CYLINDRICAL_SURFACE('',#18563,204.);
#4603=CYLINDRICAL_SURFACE('',#18564,204.);
#4604=CYLINDRICAL_SURFACE('',#18565,204.);
#4605=CYLINDRICAL_SURFACE('',#18566,204.);
#4606=CYLINDRICAL_SURFACE('',#18567,204.);
#4607=CYLINDRICAL_SURFACE('',#18568,204.);
#4608=CYLINDRICAL_SURFACE('',#18569,206.);
#4609=CYLINDRICAL_SURFACE('',#18572,145.404667636179);
#4610=CYLINDRICAL_SURFACE('',#18575,5.);
#4611=CYLINDRICAL_SURFACE('',#18577,147.404667636179);
#4612=CYLINDRICAL_SURFACE('',#18589,145.404667636179);
#4613=CYLINDRICAL_SURFACE('',#18591,206.);
#4614=CYLINDRICAL_SURFACE('',#18595,204.);
#4615=CYLINDRICAL_SURFACE('',#18596,204.);
#4616=CYLINDRICAL_SURFACE('',#18597,204.);
#4617=CYLINDRICAL_SURFACE('',#18598,204.);
#4618=CYLINDRICAL_SURFACE('',#18599,204.);
#4619=CYLINDRICAL_SURFACE('',#18600,204.);
#4620=CYLINDRICAL_SURFACE('',#18601,204.);
#4621=CYLINDRICAL_SURFACE('',#18602,204.);
#4622=CYLINDRICAL_SURFACE('',#18603,10.);
#4623=CYLINDRICAL_SURFACE('',#18606,10.);
#4624=CYLINDRICAL_SURFACE('',#18609,27.9488084273619);
#4625=CYLINDRICAL_SURFACE('',#18612,17.4625);
#4626=CYLINDRICAL_SURFACE('',#18615,25.);
#4627=CYLINDRICAL_SURFACE('',#18618,204.);
#4628=CYLINDRICAL_SURFACE('',#18621,200.);
#4629=CYLINDRICAL_SURFACE('',#18650,25.);
#4630=CYLINDRICAL_SURFACE('',#18652,25.);
#4631=CYLINDRICAL_SURFACE('',#18654,25.);
#4632=CYLINDRICAL_SURFACE('',#18656,25.);
#4633=CYLINDRICAL_SURFACE('',#18658,25.);
#4634=CYLINDRICAL_SURFACE('',#18660,25.);
#4635=CYLINDRICAL_SURFACE('',#18662,25.);
#4636=CYLINDRICAL_SURFACE('',#18664,25.);
#4637=CYLINDRICAL_SURFACE('',#18668,122.05461305459);
#4638=CYLINDRICAL_SURFACE('',#18670,77.4625);
#4639=CYLINDRICAL_SURFACE('',#18672,122.05461305459);
#4640=CYLINDRICAL_SURFACE('',#18674,122.05461305459);
#4641=CYLINDRICAL_SURFACE('',#18676,77.4625);
#4642=CYLINDRICAL_SURFACE('',#18678,122.05461305459);
#4643=CYLINDRICAL_SURFACE('',#18685,27.9488084273619);
#4644=CYLINDRICAL_SURFACE('',#18716,10.);
#4645=CYLINDRICAL_SURFACE('',#18717,10.);
#4908=FACE_OUTER_BOUND('',#5960,.T.);
#4909=FACE_OUTER_BOUND('',#5961,.T.);
#4910=FACE_OUTER_BOUND('',#5962,.T.);
#4911=FACE_OUTER_BOUND('',#5963,.T.);
#4912=FACE_OUTER_BOUND('',#5964,.T.);
#4913=FACE_OUTER_BOUND('',#5966,.T.);
#4914=FACE_OUTER_BOUND('',#5968,.T.);
#4915=FACE_OUTER_BOUND('',#5969,.T.);
#4916=FACE_OUTER_BOUND('',#5970,.T.);
#4917=FACE_OUTER_BOUND('',#5971,.T.);
#4918=FACE_OUTER_BOUND('',#5972,.T.);
#4919=FACE_OUTER_BOUND('',#5973,.T.);
#4920=FACE_OUTER_BOUND('',#5974,.T.);
#4921=FACE_OUTER_BOUND('',#5975,.T.);
#4922=FACE_OUTER_BOUND('',#5976,.T.);
#4923=FACE_OUTER_BOUND('',#5977,.T.);
#4924=FACE_OUTER_BOUND('',#5978,.T.);
#4925=FACE_OUTER_BOUND('',#5979,.T.);
#4926=FACE_OUTER_BOUND('',#5980,.T.);
#4927=FACE_OUTER_BOUND('',#5981,.T.);
#4928=FACE_OUTER_BOUND('',#5982,.T.);
#4929=FACE_OUTER_BOUND('',#5983,.T.);
#4930=FACE_OUTER_BOUND('',#5984,.T.);
#4931=FACE_OUTER_BOUND('',#5985,.T.);
#4932=FACE_OUTER_BOUND('',#5987,.T.);
#4933=FACE_OUTER_BOUND('',#5989,.T.);
#4934=FACE_OUTER_BOUND('',#5990,.T.);
#4935=FACE_OUTER_BOUND('',#5991,.T.);
#4936=FACE_OUTER_BOUND('',#5992,.T.);
#4937=FACE_OUTER_BOUND('',#5993,.T.);
#4938=FACE_OUTER_BOUND('',#5996,.T.);
#4939=FACE_OUTER_BOUND('',#5999,.T.);
#4940=FACE_OUTER_BOUND('',#6000,.T.);
#4941=FACE_OUTER_BOUND('',#6001,.T.);
#4942=FACE_OUTER_BOUND('',#6002,.T.);
#4943=FACE_OUTER_BOUND('',#6003,.T.);
#4944=FACE_OUTER_BOUND('',#6004,.T.);
#4945=FACE_OUTER_BOUND('',#6005,.T.);
#4946=FACE_OUTER_BOUND('',#6006,.T.);
#4947=FACE_OUTER_BOUND('',#6007,.T.);
#4948=FACE_OUTER_BOUND('',#6008,.T.);
#4949=FACE_OUTER_BOUND('',#6009,.T.);
#4950=FACE_OUTER_BOUND('',#6011,.T.);
#4951=FACE_OUTER_BOUND('',#6017,.T.);
#4952=FACE_OUTER_BOUND('',#6019,.T.);
#4953=FACE_OUTER_BOUND('',#6020,.T.);
#4954=FACE_OUTER_BOUND('',#6021,.T.);
#4955=FACE_OUTER_BOUND('',#6022,.T.);
#4956=FACE_OUTER_BOUND('',#6023,.T.);
#4957=FACE_OUTER_BOUND('',#6024,.T.);
#4958=FACE_OUTER_BOUND('',#6025,.T.);
#4959=FACE_OUTER_BOUND('',#6026,.T.);
#4960=FACE_OUTER_BOUND('',#6027,.T.);
#4961=FACE_OUTER_BOUND('',#6029,.T.);
#4962=FACE_OUTER_BOUND('',#6031,.T.);
#4963=FACE_OUTER_BOUND('',#6032,.T.);
#4964=FACE_OUTER_BOUND('',#6033,.T.);
#4965=FACE_OUTER_BOUND('',#6034,.T.);
#4966=FACE_OUTER_BOUND('',#6035,.T.);
#4967=FACE_OUTER_BOUND('',#6036,.T.);
#4968=FACE_OUTER_BOUND('',#6037,.T.);
#4969=FACE_OUTER_BOUND('',#6039,.T.);
#4970=FACE_OUTER_BOUND('',#6041,.T.);
#4971=FACE_OUTER_BOUND('',#6042,.T.);
#4972=FACE_OUTER_BOUND('',#6043,.T.);
#4973=FACE_OUTER_BOUND('',#6044,.T.);
#4974=FACE_OUTER_BOUND('',#6045,.T.);
#4975=FACE_OUTER_BOUND('',#6046,.T.);
#4976=FACE_OUTER_BOUND('',#6047,.T.);
#4977=FACE_OUTER_BOUND('',#6048,.T.);
#4978=FACE_OUTER_BOUND('',#6049,.T.);
#4979=FACE_OUTER_BOUND('',#6050,.T.);
#4980=FACE_OUTER_BOUND('',#6051,.T.);
#4981=FACE_OUTER_BOUND('',#6052,.T.);
#4982=FACE_OUTER_BOUND('',#6053,.T.);
#4983=FACE_OUTER_BOUND('',#6054,.T.);
#4984=FACE_OUTER_BOUND('',#6055,.T.);
#4985=FACE_OUTER_BOUND('',#6056,.T.);
#4986=FACE_OUTER_BOUND('',#6057,.T.);
#4987=FACE_OUTER_BOUND('',#6058,.T.);
#4988=FACE_OUTER_BOUND('',#6059,.T.);
#4989=FACE_OUTER_BOUND('',#6060,.T.);
#4990=FACE_OUTER_BOUND('',#6061,.T.);
#4991=FACE_OUTER_BOUND('',#6062,.T.);
#4992=FACE_OUTER_BOUND('',#6063,.T.);
#4993=FACE_OUTER_BOUND('',#6064,.T.);
#4994=FACE_OUTER_BOUND('',#6065,.T.);
#4995=FACE_OUTER_BOUND('',#6066,.T.);
#4996=FACE_OUTER_BOUND('',#6067,.T.);
#4997=FACE_OUTER_BOUND('',#6068,.T.);
#4998=FACE_OUTER_BOUND('',#6069,.T.);
#4999=FACE_OUTER_BOUND('',#6070,.T.);
#5000=FACE_OUTER_BOUND('',#6071,.T.);
#5001=FACE_OUTER_BOUND('',#6072,.T.);
#5002=FACE_OUTER_BOUND('',#6073,.T.);
#5003=FACE_OUTER_BOUND('',#6074,.T.);
#5004=FACE_OUTER_BOUND('',#6075,.T.);
#5005=FACE_OUTER_BOUND('',#6076,.T.);
#5006=FACE_OUTER_BOUND('',#6077,.T.);
#5007=FACE_OUTER_BOUND('',#6078,.T.);
#5960=EDGE_LOOP('',(#12466,#12467,#12468,#12469));
#5961=EDGE_LOOP('',(#12470,#12471,#12472,#12473));
#5962=EDGE_LOOP('',(#12474,#12475,#12476,#12477,#12478,#12479,#12480,#12481,
#12482,#12483,#12484));
#5963=EDGE_LOOP('',(#12485,#12486,#12487,#12488));
#5964=EDGE_LOOP('',(#12489,#12490));
#5965=EDGE_LOOP('',(#12491,#12492));
#5966=EDGE_LOOP('',(#12493,#12494));
#5967=EDGE_LOOP('',(#12495,#12496));
#5968=EDGE_LOOP('',(#12497));
#5969=EDGE_LOOP('',(#12498,#12499,#12500,#12501));
#5970=EDGE_LOOP('',(#12502,#12503,#12504,#12505));
#5971=EDGE_LOOP('',(#12506,#12507));
#5972=EDGE_LOOP('',(#12508,#12509));
#5973=EDGE_LOOP('',(#12510,#12511));
#5974=EDGE_LOOP('',(#12512,#12513));
#5975=EDGE_LOOP('',(#12514,#12515));
#5976=EDGE_LOOP('',(#12516,#12517));
#5977=EDGE_LOOP('',(#12518,#12519));
#5978=EDGE_LOOP('',(#12520,#12521));
#5979=EDGE_LOOP('',(#12522,#12523));
#5980=EDGE_LOOP('',(#12524,#12525));
#5981=EDGE_LOOP('',(#12526,#12527,#12528,#12529));
#5982=EDGE_LOOP('',(#12530,#12531,#12532,#12533));
#5983=EDGE_LOOP('',(#12534,#12535,#12536,#12537,#12538,#12539,#12540,#12541,
#12542,#12543,#12544));
#5984=EDGE_LOOP('',(#12545,#12546,#12547,#12548));
#5985=EDGE_LOOP('',(#12549,#12550,#12551));
#5986=EDGE_LOOP('',(#12552,#12553));
#5987=EDGE_LOOP('',(#12554,#12555,#12556));
#5988=EDGE_LOOP('',(#12557,#12558));
#5989=EDGE_LOOP('',(#12559));
#5990=EDGE_LOOP('',(#12560,#12561,#12562,#12563));
#5991=EDGE_LOOP('',(#12564,#12565,#12566,#12567));
#5992=EDGE_LOOP('',(#12568,#12569));
#5993=EDGE_LOOP('',(#12570,#12571));
#5994=EDGE_LOOP('',(#12572,#12573));
#5995=EDGE_LOOP('',(#12574,#12575));
#5996=EDGE_LOOP('',(#12576,#12577));
#5997=EDGE_LOOP('',(#12578,#12579));
#5998=EDGE_LOOP('',(#12580,#12581));
#5999=EDGE_LOOP('',(#12582,#12583));
#6000=EDGE_LOOP('',(#12584,#12585));
#6001=EDGE_LOOP('',(#12586,#12587));
#6002=EDGE_LOOP('',(#12588,#12589,#12590,#12591,#12592,#12593,#12594));
#6003=EDGE_LOOP('',(#12595,#12596,#12597,#12598));
#6004=EDGE_LOOP('',(#12599,#12600,#12601,#12602));
#6005=EDGE_LOOP('',(#12603,#12604,#12605,#12606,#12607,#12608,#12609));
#6006=EDGE_LOOP('',(#12610,#12611,#12612,#12613));
#6007=EDGE_LOOP('',(#12614,#12615,#12616,#12617));
#6008=EDGE_LOOP('',(#12618,#12619,#12620,#12621));
#6009=EDGE_LOOP('',(#12622,#12623,#12624,#12625,#12626,#12627,#12628,#12629,
#12630,#12631,#12632,#12633));
#6010=EDGE_LOOP('',(#12634,#12635,#12636,#12637));
#6011=EDGE_LOOP('',(#12638,#12639,#12640,#12641,#12642,#12643,#12644,#12645,
#12646));
#6012=EDGE_LOOP('',(#12647,#12648));
#6013=EDGE_LOOP('',(#12649,#12650,#12651,#12652));
#6014=EDGE_LOOP('',(#12653,#12654,#12655,#12656));
#6015=EDGE_LOOP('',(#12657,#12658,#12659,#12660));
#6016=EDGE_LOOP('',(#12661,#12662,#12663,#12664));
#6017=EDGE_LOOP('',(#12665,#12666,#12667,#12668,#12669,#12670,#12671,#12672,
#12673,#12674,#12675,#12676,#12677,#12678,#12679,#12680));
#6018=EDGE_LOOP('',(#12681,#12682,#12683,#12684,#12685,#12686,#12687,#12688,
#12689,#12690,#12691,#12692,#12693,#12694,#12695,#12696,#12697,#12698,#12699,
#12700,#12701,#12702,#12703,#12704,#12705,#12706,#12707,#12708,#12709,#12710,
#12711,#12712,#12713,#12714,#12715,#12716,#12717,#12718,#12719));
#6019=EDGE_LOOP('',(#12720,#12721,#12722,#12723));
#6020=EDGE_LOOP('',(#12724,#12725,#12726,#12727));
#6021=EDGE_LOOP('',(#12728,#12729,#12730,#12731));
#6022=EDGE_LOOP('',(#12732,#12733,#12734,#12735));
#6023=EDGE_LOOP('',(#12736,#12737,#12738,#12739));
#6024=EDGE_LOOP('',(#12740,#12741,#12742,#12743));
#6025=EDGE_LOOP('',(#12744,#12745,#12746,#12747));
#6026=EDGE_LOOP('',(#12748,#12749,#12750,#12751));
#6027=EDGE_LOOP('',(#12752));
#6028=EDGE_LOOP('',(#12753));
#6029=EDGE_LOOP('',(#12754));
#6030=EDGE_LOOP('',(#12755));
#6031=EDGE_LOOP('',(#12756,#12757,#12758,#12759));
#6032=EDGE_LOOP('',(#12760,#12761,#12762,#12763));
#6033=EDGE_LOOP('',(#12764,#12765,#12766,#12767));
#6034=EDGE_LOOP('',(#12768,#12769,#12770,#12771));
#6035=EDGE_LOOP('',(#12772,#12773,#12774,#12775));
#6036=EDGE_LOOP('',(#12776,#12777,#12778,#12779));
#6037=EDGE_LOOP('',(#12780,#12781,#12782,#12783,#12784,#12785,#12786,#12787,
#12788,#12789,#12790,#12791,#12792,#12793,#12794,#12795));
#6038=EDGE_LOOP('',(#12796,#12797,#12798,#12799));
#6039=EDGE_LOOP('',(#12800,#12801,#12802,#12803,#12804,#12805,#12806,#12807,
#12808,#12809,#12810,#12811,#12812,#12813,#12814,#12815,#12816,#12817,#12818,
#12819,#12820,#12821,#12822,#12823,#12824,#12825,#12826,#12827,#12828,#12829,
#12830,#12831,#12832,#12833,#12834,#12835,#12836,#12837,#12838));
#6040=EDGE_LOOP('',(#12839,#12840,#12841,#12842));
#6041=EDGE_LOOP('',(#12843,#12844,#12845,#12846));
#6042=EDGE_LOOP('',(#12847,#12848,#12849,#12850));
#6043=EDGE_LOOP('',(#12851,#12852,#12853,#12854));
#6044=EDGE_LOOP('',(#12855,#12856,#12857,#12858));
#6045=EDGE_LOOP('',(#12859,#12860,#12861,#12862));
#6046=EDGE_LOOP('',(#12863,#12864,#12865,#12866));
#6047=EDGE_LOOP('',(#12867,#12868,#12869,#12870));
#6048=EDGE_LOOP('',(#12871,#12872,#12873,#12874));
#6049=EDGE_LOOP('',(#12875,#12876,#12877,#12878));
#6050=EDGE_LOOP('',(#12879,#12880,#12881,#12882));
#6051=EDGE_LOOP('',(#12883,#12884,#12885,#12886));
#6052=EDGE_LOOP('',(#12887,#12888,#12889,#12890));
#6053=EDGE_LOOP('',(#12891,#12892,#12893,#12894));
#6054=EDGE_LOOP('',(#12895,#12896,#12897,#12898));
#6055=EDGE_LOOP('',(#12899,#12900,#12901,#12902));
#6056=EDGE_LOOP('',(#12903,#12904,#12905,#12906));
#6057=EDGE_LOOP('',(#12907,#12908,#12909,#12910));
#6058=EDGE_LOOP('',(#12911,#12912,#12913,#12914));
#6059=EDGE_LOOP('',(#12915,#12916,#12917,#12918));
#6060=EDGE_LOOP('',(#12919,#12920,#12921,#12922));
#6061=EDGE_LOOP('',(#12923,#12924,#12925,#12926));
#6062=EDGE_LOOP('',(#12927,#12928,#12929,#12930));
#6063=EDGE_LOOP('',(#12931,#12932,#12933,#12934));
#6064=EDGE_LOOP('',(#12935,#12936,#12937,#12938));
#6065=EDGE_LOOP('',(#12939,#12940,#12941,#12942));
#6066=EDGE_LOOP('',(#12943,#12944,#12945,#12946));
#6067=EDGE_LOOP('',(#12947,#12948,#12949,#12950));
#6068=EDGE_LOOP('',(#12951,#12952,#12953,#12954));
#6069=EDGE_LOOP('',(#12955,#12956,#12957,#12958));
#6070=EDGE_LOOP('',(#12959,#12960,#12961,#12962));
#6071=EDGE_LOOP('',(#12963,#12964,#12965,#12966));
#6072=EDGE_LOOP('',(#12967,#12968,#12969,#12970,#12971,#12972,#12973,#12974));
#6073=EDGE_LOOP('',(#12975,#12976,#12977,#12978));
#6074=EDGE_LOOP('',(#12979,#12980,#12981,#12982));
#6075=EDGE_LOOP('',(#12983,#12984,#12985,#12986,#12987,#12988,#12989));
#6076=EDGE_LOOP('',(#12990,#12991,#12992,#12993));
#6077=EDGE_LOOP('',(#12994,#12995,#12996,#12997));
#6078=EDGE_LOOP('',(#12998,#12999,#13000,#13001));
#7087=CIRCLE('',#18538,206.);
#7088=CIRCLE('',#18539,206.);
#7089=CIRCLE('',#18541,145.404667636179);
#7090=CIRCLE('',#18542,145.404667636179);
#7091=CIRCLE('',#18544,5.);
#7092=CIRCLE('',#18546,147.404667636179);
#7093=CIRCLE('',#18547,147.404667636179);
#7094=CIRCLE('',#18549,204.);
#7095=CIRCLE('',#18551,204.);
#7096=CIRCLE('',#18552,145.404667636179);
#7097=CIRCLE('',#18553,206.);
#7098=CIRCLE('',#18556,145.404667636179);
#7099=CIRCLE('',#18558,206.);
#7100=CIRCLE('',#18570,206.);
#7101=CIRCLE('',#18571,206.);
#7102=CIRCLE('',#18573,145.404667636179);
#7103=CIRCLE('',#18574,145.404667636179);
#7104=CIRCLE('',#18576,5.);
#7105=CIRCLE('',#18578,147.404667636179);
#7106=CIRCLE('',#18579,147.404667636179);
#7107=CIRCLE('',#18581,204.);
#7108=CIRCLE('',#18582,204.);
#7109=CIRCLE('',#18584,204.);
#7110=CIRCLE('',#18585,204.);
#7111=CIRCLE('',#18586,145.404667636179);
#7112=CIRCLE('',#18587,206.);
#7113=CIRCLE('',#18590,145.404667636179);
#7114=CIRCLE('',#18592,206.);
#7115=CIRCLE('',#18604,10.);
#7116=CIRCLE('',#18605,10.);
#7117=CIRCLE('',#18607,10.);
#7118=CIRCLE('',#18608,10.);
#7119=CIRCLE('',#18610,27.9488084273619);
#7120=CIRCLE('',#18611,27.9488084273619);
#7121=CIRCLE('',#18613,17.4625);
#7122=CIRCLE('',#18614,17.4625);
#7123=CIRCLE('',#18616,25.);
#7124=CIRCLE('',#18617,25.);
#7125=CIRCLE('',#18619,204.);
#7126=CIRCLE('',#18620,204.);
#7127=CIRCLE('',#18622,200.);
#7128=CIRCLE('',#18623,200.);
#7129=CIRCLE('',#18624,200.);
#7130=CIRCLE('',#18625,200.);
#7131=CIRCLE('',#18626,200.);
#7132=CIRCLE('',#18627,200.);
#7133=CIRCLE('',#18628,200.);
#7134=CIRCLE('',#18629,200.);
#7135=CIRCLE('',#18630,200.);
#7136=CIRCLE('',#18631,200.);
#7137=CIRCLE('',#18633,10.);
#7138=CIRCLE('',#18634,122.05461305459);
#7139=CIRCLE('',#18635,77.4625);
#7140=CIRCLE('',#18636,122.05461305459);
#7141=CIRCLE('',#18637,27.9488084273619);
#7142=CIRCLE('',#18638,122.05461305459);
#7143=CIRCLE('',#18639,77.4625);
#7144=CIRCLE('',#18640,122.05461305459);
#7145=CIRCLE('',#18641,10.);
#7146=CIRCLE('',#18642,25.);
#7147=CIRCLE('',#18643,25.);
#7148=CIRCLE('',#18644,25.);
#7149=CIRCLE('',#18645,25.);
#7150=CIRCLE('',#18646,25.);
#7151=CIRCLE('',#18647,25.);
#7152=CIRCLE('',#18648,25.);
#7153=CIRCLE('',#18649,25.);
#7154=CIRCLE('',#18651,25.);
#7155=CIRCLE('',#18653,25.);
#7156=CIRCLE('',#18655,25.);
#7157=CIRCLE('',#18657,25.);
#7158=CIRCLE('',#18659,25.);
#7159=CIRCLE('',#18661,25.);
#7160=CIRCLE('',#18663,25.);
#7161=CIRCLE('',#18665,25.);
#7162=CIRCLE('',#18669,122.05461305459);
#7163=CIRCLE('',#18671,77.4625);
#7164=CIRCLE('',#18673,122.05461305459);
#7165=CIRCLE('',#18675,122.05461305459);
#7166=CIRCLE('',#18677,77.4625);
#7167=CIRCLE('',#18679,122.05461305459);
#7168=CIRCLE('',#18681,10.);
#7169=CIRCLE('',#18682,27.9488084273619);
#7170=CIRCLE('',#18683,10.);
#7829=VERTEX_POINT('',#25630);
#7830=VERTEX_POINT('',#25631);
#7831=VERTEX_POINT('',#25633);
#7832=VERTEX_POINT('',#25635);
#7833=VERTEX_POINT('',#25642);
#7834=VERTEX_POINT('',#25644);
#7835=VERTEX_POINT('',#25646);
#7836=VERTEX_POINT('',#25653);
#7837=VERTEX_POINT('',#25660);
#7838=VERTEX_POINT('',#25670);
#7839=VERTEX_POINT('',#25679);
#7840=VERTEX_POINT('',#25686);
#7841=VERTEX_POINT('',#25695);
#7842=VERTEX_POINT('',#25713);
#7843=VERTEX_POINT('',#25714);
#7844=VERTEX_POINT('',#25716);
#7845=VERTEX_POINT('',#25718);
#7846=VERTEX_POINT('',#25725);
#7847=VERTEX_POINT('',#25726);
#7848=VERTEX_POINT('',#25731);
#7849=VERTEX_POINT('',#25733);
#7850=VERTEX_POINT('',#26141);
#7851=VERTEX_POINT('',#26142);
#7852=VERTEX_POINT('',#26144);
#7853=VERTEX_POINT('',#26146);
#7854=VERTEX_POINT('',#26153);
#7855=VERTEX_POINT('',#26155);
#7856=VERTEX_POINT('',#26157);
#7857=VERTEX_POINT('',#26166);
#7858=VERTEX_POINT('',#26175);
#7859=VERTEX_POINT('',#26182);
#7860=VERTEX_POINT('',#26189);
#7861=VERTEX_POINT('',#26198);
#7862=VERTEX_POINT('',#26208);
#7863=VERTEX_POINT('',#26224);
#7864=VERTEX_POINT('',#26225);
#7865=VERTEX_POINT('',#26227);
#7866=VERTEX_POINT('',#26229);
#7867=VERTEX_POINT('',#26233);
#7868=VERTEX_POINT('',#26237);
#7869=VERTEX_POINT('',#26240);
#7870=VERTEX_POINT('',#26241);
#7871=VERTEX_POINT('',#26246);
#7872=VERTEX_POINT('',#26248);
#7873=VERTEX_POINT('',#26317);
#7874=VERTEX_POINT('',#26319);
#7875=VERTEX_POINT('',#26346);
#7876=VERTEX_POINT('',#26347);
#7877=VERTEX_POINT('',#26349);
#7878=VERTEX_POINT('',#26351);
#7879=VERTEX_POINT('',#26355);
#7880=VERTEX_POINT('',#26356);
#7881=VERTEX_POINT('',#26358);
#7882=VERTEX_POINT('',#26360);
#7883=VERTEX_POINT('',#26387);
#7884=VERTEX_POINT('',#26389);
#7885=VERTEX_POINT('',#26564);
#7886=VERTEX_POINT('',#26565);
#7887=VERTEX_POINT('',#26567);
#7888=VERTEX_POINT('',#26569);
#7889=VERTEX_POINT('',#26573);
#7890=VERTEX_POINT('',#26574);
#7891=VERTEX_POINT('',#26576);
#7892=VERTEX_POINT('',#26578);
#7893=VERTEX_POINT('',#26582);
#7894=VERTEX_POINT('',#26583);
#7895=VERTEX_POINT('',#26585);
#7896=VERTEX_POINT('',#26587);
#7897=VERTEX_POINT('',#26591);
#7898=VERTEX_POINT('',#26594);
#7899=VERTEX_POINT('',#26598);
#7900=VERTEX_POINT('',#26601);
#7901=VERTEX_POINT('',#26606);
#7902=VERTEX_POINT('',#26805);
#7903=VERTEX_POINT('',#26807);
#7904=VERTEX_POINT('',#26810);
#7905=VERTEX_POINT('',#26811);
#7906=VERTEX_POINT('',#26815);
#7907=VERTEX_POINT('',#26817);
#7908=VERTEX_POINT('',#26820);
#7909=VERTEX_POINT('',#26822);
#7910=VERTEX_POINT('',#26826);
#7911=VERTEX_POINT('',#26828);
#7912=VERTEX_POINT('',#26830);
#7913=VERTEX_POINT('',#26834);
#7914=VERTEX_POINT('',#26836);
#7915=VERTEX_POINT('',#26838);
#7916=VERTEX_POINT('',#26841);
#7917=VERTEX_POINT('',#26842);
#7918=VERTEX_POINT('',#26844);
#7919=VERTEX_POINT('',#26846);
#7920=VERTEX_POINT('',#26848);
#7921=VERTEX_POINT('',#26850);
#7922=VERTEX_POINT('',#26853);
#7923=VERTEX_POINT('',#26855);
#7924=VERTEX_POINT('',#26857);
#7925=VERTEX_POINT('',#26859);
#7926=VERTEX_POINT('',#26861);
#7927=VERTEX_POINT('',#26863);
#7928=VERTEX_POINT('',#26865);
#7929=VERTEX_POINT('',#26867);
#7930=VERTEX_POINT('',#26869);
#7931=VERTEX_POINT('',#26871);
#7932=VERTEX_POINT('',#26873);
#7933=VERTEX_POINT('',#26875);
#7934=VERTEX_POINT('',#26877);
#7935=VERTEX_POINT('',#26879);
#7936=VERTEX_POINT('',#26881);
#7937=VERTEX_POINT('',#26883);
#7938=VERTEX_POINT('',#26885);
#7939=VERTEX_POINT('',#26887);
#7940=VERTEX_POINT('',#26889);
#7941=VERTEX_POINT('',#26891);
#7942=VERTEX_POINT('',#26893);
#7943=VERTEX_POINT('',#26895);
#7944=VERTEX_POINT('',#26897);
#7945=VERTEX_POINT('',#26899);
#7946=VERTEX_POINT('',#26901);
#7947=VERTEX_POINT('',#26903);
#7948=VERTEX_POINT('',#26905);
#7949=VERTEX_POINT('',#26907);
#7950=VERTEX_POINT('',#26909);
#7951=VERTEX_POINT('',#26911);
#7952=VERTEX_POINT('',#26913);
#7953=VERTEX_POINT('',#26917);
#7954=VERTEX_POINT('',#26919);
#7955=VERTEX_POINT('',#26923);
#7956=VERTEX_POINT('',#26925);
#7957=VERTEX_POINT('',#26929);
#7958=VERTEX_POINT('',#26931);
#7959=VERTEX_POINT('',#26935);
#7960=VERTEX_POINT('',#26937);
#7961=VERTEX_POINT('',#26941);
#7962=VERTEX_POINT('',#26943);
#7963=VERTEX_POINT('',#26947);
#7964=VERTEX_POINT('',#26949);
#7965=VERTEX_POINT('',#26953);
#7966=VERTEX_POINT('',#26955);
#7967=VERTEX_POINT('',#26959);
#7968=VERTEX_POINT('',#26961);
#7969=VERTEX_POINT('',#26967);
#7970=VERTEX_POINT('',#26969);
#7971=VERTEX_POINT('',#26973);
#7972=VERTEX_POINT('',#26979);
#7973=VERTEX_POINT('',#26983);
#7974=VERTEX_POINT('',#26987);
#7975=VERTEX_POINT('',#26994);
#7976=VERTEX_POINT('',#26996);
#7977=VERTEX_POINT('',#27000);
#7978=VERTEX_POINT('',#27002);
#7979=VERTEX_POINT('',#27005);
#7980=VERTEX_POINT('',#27007);
#7981=VERTEX_POINT('',#27010);
#7982=VERTEX_POINT('',#27012);
#7983=VERTEX_POINT('',#27015);
#7984=VERTEX_POINT('',#27017);
#7985=VERTEX_POINT('',#27019);
#7986=VERTEX_POINT('',#27021);
#7987=VERTEX_POINT('',#27024);
#7988=VERTEX_POINT('',#27026);
#7989=VERTEX_POINT('',#27028);
#7990=VERTEX_POINT('',#27031);
#7991=VERTEX_POINT('',#27033);
#7992=VERTEX_POINT('',#27036);
#7993=VERTEX_POINT('',#27038);
#7994=VERTEX_POINT('',#27041);
#7995=VERTEX_POINT('',#27043);
#7996=VERTEX_POINT('',#27046);
#7997=VERTEX_POINT('',#27048);
#7998=VERTEX_POINT('',#27051);
#7999=VERTEX_POINT('',#27053);
#9613=EDGE_CURVE('',#7829,#7830,#7087,.T.);
#9614=EDGE_CURVE('',#7830,#7831,#1535,.T.);
#9615=EDGE_CURVE('',#7832,#7831,#7088,.T.);
#9616=EDGE_CURVE('',#7829,#7832,#1536,.T.);
#9617=EDGE_CURVE('',#7830,#7829,#7089,.T.);
#9618=EDGE_CURVE('',#7831,#7832,#7090,.T.);
#9619=EDGE_CURVE('',#7833,#7833,#7091,.T.);
#9620=EDGE_CURVE('',#7833,#7834,#1537,.T.);
#9621=EDGE_CURVE('',#7835,#7834,#1069,.T.);
#9622=EDGE_CURVE('',#7836,#7835,#1070,.T.);
#9623=EDGE_CURVE('',#7837,#7836,#1071,.T.);
#9624=EDGE_CURVE('',#7838,#7837,#1072,.T.);
#9625=EDGE_CURVE('',#7839,#7838,#1073,.T.);
#9626=EDGE_CURVE('',#7840,#7839,#1074,.T.);
#9627=EDGE_CURVE('',#7841,#7840,#1075,.T.);
#9628=EDGE_CURVE('',#7834,#7841,#1076,.T.);
#9629=EDGE_CURVE('',#7842,#7843,#7092,.T.);
#9630=EDGE_CURVE('',#7844,#7842,#1538,.T.);
#9631=EDGE_CURVE('',#7844,#7845,#7093,.T.);
#9632=EDGE_CURVE('',#7843,#7845,#1539,.T.);
#9633=EDGE_CURVE('',#7845,#7844,#7094,.T.);
#9634=EDGE_CURVE('',#7842,#7843,#7095,.T.);
#9635=EDGE_CURVE('',#7846,#7847,#7096,.T.);
#9636=EDGE_CURVE('',#7847,#7846,#7097,.T.);
#9637=EDGE_CURVE('',#7848,#7847,#1540,.T.);
#9638=EDGE_CURVE('',#7849,#7848,#7098,.T.);
#9639=EDGE_CURVE('',#7849,#7846,#1541,.T.);
#9640=EDGE_CURVE('',#7848,#7849,#7099,.T.);
#9641=EDGE_CURVE('',#7835,#7836,#1077,.T.);
#9642=EDGE_CURVE('',#7834,#7835,#1078,.T.);
#9643=EDGE_CURVE('',#7841,#7834,#1079,.T.);
#9644=EDGE_CURVE('',#7840,#7841,#1080,.T.);
#9645=EDGE_CURVE('',#7839,#7840,#1081,.T.);
#9646=EDGE_CURVE('',#7838,#7839,#1082,.T.);
#9647=EDGE_CURVE('',#7837,#7838,#1083,.T.);
#9648=EDGE_CURVE('',#7836,#7837,#1084,.T.);
#9649=EDGE_CURVE('',#7850,#7851,#7100,.T.);
#9650=EDGE_CURVE('',#7851,#7852,#1542,.T.);
#9651=EDGE_CURVE('',#7853,#7852,#7101,.T.);
#9652=EDGE_CURVE('',#7850,#7853,#1543,.T.);
#9653=EDGE_CURVE('',#7851,#7850,#7102,.T.);
#9654=EDGE_CURVE('',#7852,#7853,#7103,.T.);
#9655=EDGE_CURVE('',#7854,#7854,#7104,.T.);
#9656=EDGE_CURVE('',#7854,#7855,#1544,.T.);
#9657=EDGE_CURVE('',#7856,#7855,#1085,.T.);
#9658=EDGE_CURVE('',#7857,#7856,#1086,.T.);
#9659=EDGE_CURVE('',#7858,#7857,#1087,.T.);
#9660=EDGE_CURVE('',#7859,#7858,#1088,.T.);
#9661=EDGE_CURVE('',#7860,#7859,#1089,.T.);
#9662=EDGE_CURVE('',#7861,#7860,#1090,.T.);
#9663=EDGE_CURVE('',#7862,#7861,#1091,.T.);
#9664=EDGE_CURVE('',#7855,#7862,#1092,.T.);
#9665=EDGE_CURVE('',#7863,#7864,#7105,.T.);
#9666=EDGE_CURVE('',#7865,#7863,#1545,.T.);
#9667=EDGE_CURVE('',#7865,#7866,#7106,.T.);
#9668=EDGE_CURVE('',#7864,#7866,#1546,.T.);
#9669=EDGE_CURVE('',#7866,#7867,#7107,.T.);
#9670=EDGE_CURVE('',#7867,#7865,#7108,.T.);
#9671=EDGE_CURVE('',#7863,#7868,#7109,.T.);
#9672=EDGE_CURVE('',#7868,#7864,#7110,.T.);
#9673=EDGE_CURVE('',#7869,#7870,#7111,.T.);
#9674=EDGE_CURVE('',#7870,#7869,#7112,.T.);
#9675=EDGE_CURVE('',#7871,#7870,#1547,.T.);
#9676=EDGE_CURVE('',#7872,#7871,#7113,.T.);
#9677=EDGE_CURVE('',#7872,#7869,#1548,.T.);
#9678=EDGE_CURVE('',#7871,#7872,#7114,.T.);
#9679=EDGE_CURVE('',#7860,#7859,#1093,.T.);
#9680=EDGE_CURVE('',#7859,#7858,#1094,.T.);
#9681=EDGE_CURVE('',#7858,#7857,#1095,.T.);
#9682=EDGE_CURVE('',#7857,#7856,#1096,.T.);
#9683=EDGE_CURVE('',#7856,#7855,#1097,.T.);
#9684=EDGE_CURVE('',#7855,#7862,#1098,.T.);
#9685=EDGE_CURVE('',#7862,#7861,#1099,.T.);
#9686=EDGE_CURVE('',#7861,#7860,#1100,.T.);
#9687=EDGE_CURVE('',#7838,#7873,#1549,.T.);
#9688=EDGE_CURVE('',#7873,#7874,#1101,.T.);
#9689=EDGE_CURVE('',#7834,#7874,#1550,.T.);
#9690=EDGE_CURVE('',#7875,#7876,#7115,.T.);
#9691=EDGE_CURVE('',#7877,#7875,#1551,.T.);
#9692=EDGE_CURVE('',#7878,#7877,#7116,.T.);
#9693=EDGE_CURVE('',#7876,#7878,#1552,.T.);
#9694=EDGE_CURVE('',#7879,#7880,#7117,.T.);
#9695=EDGE_CURVE('',#7881,#7879,#1553,.T.);
#9696=EDGE_CURVE('',#7882,#7881,#7118,.T.);
#9697=EDGE_CURVE('',#7880,#7882,#1554,.T.);
#9698=EDGE_CURVE('',#7855,#7883,#1555,.T.);
#9699=EDGE_CURVE('',#7884,#7883,#1102,.T.);
#9700=EDGE_CURVE('',#7859,#7884,#1556,.T.);
#9701=EDGE_CURVE('',#7885,#7886,#7119,.T.);
#9702=EDGE_CURVE('',#7885,#7887,#1557,.T.);
#9703=EDGE_CURVE('',#7887,#7888,#7120,.T.);
#9704=EDGE_CURVE('',#7886,#7888,#1558,.T.);
#9705=EDGE_CURVE('',#7889,#7890,#7121,.T.);
#9706=EDGE_CURVE('',#7890,#7891,#1559,.T.);
#9707=EDGE_CURVE('',#7891,#7892,#7122,.T.);
#9708=EDGE_CURVE('',#7892,#7889,#1560,.T.);
#9709=EDGE_CURVE('',#7893,#7894,#7123,.T.);
#9710=EDGE_CURVE('',#7894,#7895,#1561,.T.);
#9711=EDGE_CURVE('',#7896,#7895,#7124,.T.);
#9712=EDGE_CURVE('',#7893,#7896,#1562,.T.);
#9713=EDGE_CURVE('',#7897,#7897,#7125,.T.);
#9714=EDGE_CURVE('',#7897,#7868,#1563,.T.);
#9715=EDGE_CURVE('',#7867,#7898,#1564,.T.);
#9716=EDGE_CURVE('',#7898,#7898,#7126,.T.);
#9717=EDGE_CURVE('',#7899,#7899,#7127,.T.);
#9718=EDGE_CURVE('',#7899,#7884,#1565,.T.);
#9719=EDGE_CURVE('',#7883,#7900,#1103,.F.);
#9720=EDGE_CURVE('',#7900,#7901,#1566,.T.);
#9721=EDGE_CURVE('',#7901,#7901,#7128,.T.);
#9722=EDGE_CURVE('',#7900,#7884,#1104,.F.);
#9723=EDGE_CURVE('',#7874,#7873,#1105,.T.);
#9724=EDGE_CURVE('',#7902,#7876,#7129,.T.);
#9725=EDGE_CURVE('',#7903,#7878,#7130,.T.);
#9726=EDGE_CURVE('',#7902,#7903,#1567,.T.);
#9727=EDGE_CURVE('',#7904,#7905,#1568,.T.);
#9728=EDGE_CURVE('',#7905,#7886,#7131,.T.);
#9729=EDGE_CURVE('',#7904,#7888,#7132,.T.);
#9730=EDGE_CURVE('',#7885,#7906,#7133,.T.);
#9731=EDGE_CURVE('',#7906,#7907,#1569,.T.);
#9732=EDGE_CURVE('',#7887,#7907,#7134,.T.);
#9733=EDGE_CURVE('',#7879,#7908,#7135,.T.);
#9734=EDGE_CURVE('',#7908,#7909,#1570,.T.);
#9735=EDGE_CURVE('',#7881,#7909,#7136,.T.);
#9736=EDGE_CURVE('',#7907,#7910,#7137,.T.);
#9737=EDGE_CURVE('',#7910,#7911,#7138,.T.);
#9738=EDGE_CURVE('',#7911,#7912,#7139,.T.);
#9739=EDGE_CURVE('',#7882,#7912,#7140,.T.);
#9740=EDGE_CURVE('',#7903,#7909,#7141,.T.);
#9741=EDGE_CURVE('',#7877,#7913,#7142,.T.);
#9742=EDGE_CURVE('',#7913,#7914,#7143,.T.);
#9743=EDGE_CURVE('',#7915,#7914,#7144,.T.);
#9744=EDGE_CURVE('',#7915,#7904,#7145,.T.);
#9745=EDGE_CURVE('',#7916,#7917,#1571,.T.);
#9746=EDGE_CURVE('',#7918,#7916,#1572,.T.);
#9747=EDGE_CURVE('',#7919,#7918,#7146,.T.);
#9748=EDGE_CURVE('',#7919,#7920,#1573,.T.);
#9749=EDGE_CURVE('',#7921,#7920,#1574,.T.);
#9750=EDGE_CURVE('',#7894,#7921,#1575,.T.);
#9751=EDGE_CURVE('',#7893,#7922,#1576,.T.);
#9752=EDGE_CURVE('',#7923,#7922,#1577,.T.);
#9753=EDGE_CURVE('',#7924,#7923,#1578,.T.);
#9754=EDGE_CURVE('',#7925,#7924,#7147,.T.);
#9755=EDGE_CURVE('',#7925,#7926,#1579,.T.);
#9756=EDGE_CURVE('',#7927,#7926,#1580,.T.);
#9757=EDGE_CURVE('',#7928,#7927,#1581,.T.);
#9758=EDGE_CURVE('',#7929,#7928,#7148,.T.);
#9759=EDGE_CURVE('',#7929,#7930,#1582,.T.);
#9760=EDGE_CURVE('',#7931,#7930,#1583,.T.);
#9761=EDGE_CURVE('',#7932,#7931,#1584,.T.);
#9762=EDGE_CURVE('',#7933,#7932,#7149,.T.);
#9763=EDGE_CURVE('',#7933,#7934,#1585,.T.);
#9764=EDGE_CURVE('',#7935,#7934,#1586,.T.);
#9765=EDGE_CURVE('',#7936,#7935,#1587,.T.);
#9766=EDGE_CURVE('',#7936,#7937,#1588,.T.);
#9767=EDGE_CURVE('',#7938,#7937,#7150,.T.);
#9768=EDGE_CURVE('',#7938,#7939,#1589,.T.);
#9769=EDGE_CURVE('',#7939,#7940,#1590,.T.);
#9770=EDGE_CURVE('',#7941,#7940,#1591,.T.);
#9771=EDGE_CURVE('',#7942,#7941,#1592,.T.);
#9772=EDGE_CURVE('',#7942,#7943,#1593,.T.);
#9773=EDGE_CURVE('',#7944,#7943,#7151,.T.);
#9774=EDGE_CURVE('',#7944,#7945,#1594,.T.);
#9775=EDGE_CURVE('',#7946,#7945,#1595,.T.);
#9776=EDGE_CURVE('',#7947,#7946,#1596,.T.);
#9777=EDGE_CURVE('',#7948,#7947,#7152,.T.);
#9778=EDGE_CURVE('',#7948,#7949,#1597,.T.);
#9779=EDGE_CURVE('',#7950,#7949,#1598,.T.);
#9780=EDGE_CURVE('',#7951,#7950,#1599,.T.);
#9781=EDGE_CURVE('',#7952,#7951,#7153,.T.);
#9782=EDGE_CURVE('',#7952,#7917,#1600,.T.);
#9783=EDGE_CURVE('',#7918,#7953,#1601,.T.);
#9784=EDGE_CURVE('',#7954,#7953,#7154,.T.);
#9785=EDGE_CURVE('',#7919,#7954,#1602,.T.);
#9786=EDGE_CURVE('',#7924,#7955,#1603,.T.);
#9787=EDGE_CURVE('',#7956,#7955,#7155,.T.);
#9788=EDGE_CURVE('',#7925,#7956,#1604,.T.);
#9789=EDGE_CURVE('',#7928,#7957,#1605,.T.);
#9790=EDGE_CURVE('',#7958,#7957,#7156,.T.);
#9791=EDGE_CURVE('',#7929,#7958,#1606,.T.);
#9792=EDGE_CURVE('',#7932,#7959,#1607,.T.);
#9793=EDGE_CURVE('',#7960,#7959,#7157,.T.);
#9794=EDGE_CURVE('',#7933,#7960,#1608,.T.);
#9795=EDGE_CURVE('',#7937,#7961,#1609,.T.);
#9796=EDGE_CURVE('',#7962,#7961,#7158,.T.);
#9797=EDGE_CURVE('',#7962,#7938,#1610,.T.);
#9798=EDGE_CURVE('',#7952,#7963,#1611,.T.);
#9799=EDGE_CURVE('',#7951,#7964,#1612,.T.);
#9800=EDGE_CURVE('',#7963,#7964,#7159,.T.);
#9801=EDGE_CURVE('',#7943,#7965,#1613,.T.);
#9802=EDGE_CURVE('',#7966,#7965,#7160,.T.);
#9803=EDGE_CURVE('',#7944,#7966,#1614,.T.);
#9804=EDGE_CURVE('',#7947,#7967,#1615,.T.);
#9805=EDGE_CURVE('',#7968,#7967,#7161,.T.);
#9806=EDGE_CURVE('',#7948,#7968,#1616,.T.);
#9807=EDGE_CURVE('',#7910,#7969,#1617,.T.);
#9808=EDGE_CURVE('',#7969,#7970,#7162,.T.);
#9809=EDGE_CURVE('',#7911,#7970,#1618,.T.);
#9810=EDGE_CURVE('',#7970,#7971,#7163,.T.);
#9811=EDGE_CURVE('',#7912,#7971,#1619,.T.);
#9812=EDGE_CURVE('',#7880,#7971,#7164,.T.);
#9813=EDGE_CURVE('',#7875,#7972,#7165,.T.);
#9814=EDGE_CURVE('',#7913,#7972,#1620,.T.);
#9815=EDGE_CURVE('',#7972,#7973,#7166,.T.);
#9816=EDGE_CURVE('',#7914,#7973,#1621,.T.);
#9817=EDGE_CURVE('',#7974,#7973,#7167,.T.);
#9818=EDGE_CURVE('',#7974,#7915,#1622,.T.);
#9819=EDGE_CURVE('',#7905,#7974,#7168,.T.);
#9820=EDGE_CURVE('',#7902,#7908,#7169,.T.);
#9821=EDGE_CURVE('',#7969,#7906,#7170,.T.);
#9822=EDGE_CURVE('',#7889,#7975,#1623,.T.);
#9823=EDGE_CURVE('',#7975,#7976,#1624,.T.);
#9824=EDGE_CURVE('',#7976,#7890,#1625,.T.);
#9825=EDGE_CURVE('',#7977,#7953,#1626,.T.);
#9826=EDGE_CURVE('',#7977,#7978,#1627,.T.);
#9827=EDGE_CURVE('',#7978,#7963,#1628,.T.);
#9828=EDGE_CURVE('',#7979,#7964,#1629,.T.);
#9829=EDGE_CURVE('',#7979,#7980,#1630,.T.);
#9830=EDGE_CURVE('',#7980,#7968,#1631,.T.);
#9831=EDGE_CURVE('',#7981,#7967,#1632,.T.);
#9832=EDGE_CURVE('',#7981,#7982,#1633,.T.);
#9833=EDGE_CURVE('',#7982,#7966,#1634,.T.);
#9834=EDGE_CURVE('',#7983,#7965,#1635,.T.);
#9835=EDGE_CURVE('',#7984,#7983,#1636,.T.);
#9836=EDGE_CURVE('',#7984,#7985,#1637,.T.);
#9837=EDGE_CURVE('',#7985,#7986,#1638,.T.);
#9838=EDGE_CURVE('',#7962,#7986,#1639,.T.);
#9839=EDGE_CURVE('',#7987,#7961,#1640,.T.);
#9840=EDGE_CURVE('',#7988,#7987,#1641,.T.);
#9841=EDGE_CURVE('',#7988,#7989,#1642,.T.);
#9842=EDGE_CURVE('',#7989,#7960,#1643,.T.);
#9843=EDGE_CURVE('',#7990,#7959,#1644,.T.);
#9844=EDGE_CURVE('',#7990,#7991,#1645,.T.);
#9845=EDGE_CURVE('',#7991,#7958,#1646,.T.);
#9846=EDGE_CURVE('',#7992,#7957,#1647,.T.);
#9847=EDGE_CURVE('',#7992,#7993,#1648,.T.);
#9848=EDGE_CURVE('',#7993,#7956,#1649,.T.);
#9849=EDGE_CURVE('',#7994,#7955,#1650,.T.);
#9850=EDGE_CURVE('',#7994,#7995,#1651,.T.);
#9851=EDGE_CURVE('',#7995,#7896,#1652,.T.);
#9852=EDGE_CURVE('',#7996,#7895,#1653,.T.);
#9853=EDGE_CURVE('',#7996,#7997,#1654,.T.);
#9854=EDGE_CURVE('',#7997,#7954,#1655,.T.);
#9855=EDGE_CURVE('',#7892,#7998,#1656,.T.);
#9856=EDGE_CURVE('',#7999,#7891,#1657,.T.);
#9857=EDGE_CURVE('',#7998,#7999,#1658,.T.);
#9858=EDGE_CURVE('',#7949,#7980,#1659,.T.);
#9859=EDGE_CURVE('',#7950,#7979,#1660,.T.);
#9860=EDGE_CURVE('',#7945,#7982,#1661,.T.);
#9861=EDGE_CURVE('',#7946,#7981,#1662,.T.);
#9862=EDGE_CURVE('',#7986,#7939,#1663,.T.);
#9863=EDGE_CURVE('',#7983,#7942,#1664,.T.);
#9864=EDGE_CURVE('',#7940,#7985,#1665,.T.);
#9865=EDGE_CURVE('',#7941,#7984,#1666,.T.);
#9866=EDGE_CURVE('',#7987,#7936,#1667,.T.);
#9867=EDGE_CURVE('',#7934,#7989,#1668,.T.);
#9868=EDGE_CURVE('',#7935,#7988,#1669,.T.);
#9869=EDGE_CURVE('',#7930,#7991,#1670,.T.);
#9870=EDGE_CURVE('',#7931,#7990,#1671,.T.);
#9871=EDGE_CURVE('',#7926,#7993,#1672,.T.);
#9872=EDGE_CURVE('',#7927,#7992,#1673,.T.);
#9873=EDGE_CURVE('',#7922,#7995,#1674,.T.);
#9874=EDGE_CURVE('',#7923,#7994,#1675,.T.);
#9875=EDGE_CURVE('',#7920,#7997,#1676,.T.);
#9876=EDGE_CURVE('',#7921,#7996,#1677,.T.);
#9877=EDGE_CURVE('',#7917,#7978,#1678,.T.);
#9878=EDGE_CURVE('',#7916,#7977,#1679,.T.);
#9879=EDGE_CURVE('',#7975,#7998,#1680,.T.);
#9880=EDGE_CURVE('',#7976,#7999,#1681,.T.);
#12466=ORIENTED_EDGE('',*,*,#9613,.T.);
#12467=ORIENTED_EDGE('',*,*,#9614,.T.);
#12468=ORIENTED_EDGE('',*,*,#9615,.F.);
#12469=ORIENTED_EDGE('',*,*,#9616,.F.);
#12470=ORIENTED_EDGE('',*,*,#9617,.T.);
#12471=ORIENTED_EDGE('',*,*,#9616,.T.);
#12472=ORIENTED_EDGE('',*,*,#9618,.F.);
#12473=ORIENTED_EDGE('',*,*,#9614,.F.);
#12474=ORIENTED_EDGE('',*,*,#9619,.F.);
#12475=ORIENTED_EDGE('',*,*,#9620,.T.);
#12476=ORIENTED_EDGE('',*,*,#9621,.F.);
#12477=ORIENTED_EDGE('',*,*,#9622,.F.);
#12478=ORIENTED_EDGE('',*,*,#9623,.F.);
#12479=ORIENTED_EDGE('',*,*,#9624,.F.);
#12480=ORIENTED_EDGE('',*,*,#9625,.F.);
#12481=ORIENTED_EDGE('',*,*,#9626,.F.);
#12482=ORIENTED_EDGE('',*,*,#9627,.F.);
#12483=ORIENTED_EDGE('',*,*,#9628,.F.);
#12484=ORIENTED_EDGE('',*,*,#9620,.F.);
#12485=ORIENTED_EDGE('',*,*,#9629,.F.);
#12486=ORIENTED_EDGE('',*,*,#9630,.F.);
#12487=ORIENTED_EDGE('',*,*,#9631,.T.);
#12488=ORIENTED_EDGE('',*,*,#9632,.F.);
#12489=ORIENTED_EDGE('',*,*,#9633,.F.);
#12490=ORIENTED_EDGE('',*,*,#9631,.F.);
#12491=ORIENTED_EDGE('',*,*,#9618,.T.);
#12492=ORIENTED_EDGE('',*,*,#9615,.T.);
#12493=ORIENTED_EDGE('',*,*,#9634,.F.);
#12494=ORIENTED_EDGE('',*,*,#9629,.T.);
#12495=ORIENTED_EDGE('',*,*,#9635,.F.);
#12496=ORIENTED_EDGE('',*,*,#9636,.F.);
#12497=ORIENTED_EDGE('',*,*,#9619,.T.);
#12498=ORIENTED_EDGE('',*,*,#9635,.T.);
#12499=ORIENTED_EDGE('',*,*,#9637,.F.);
#12500=ORIENTED_EDGE('',*,*,#9638,.F.);
#12501=ORIENTED_EDGE('',*,*,#9639,.T.);
#12502=ORIENTED_EDGE('',*,*,#9636,.T.);
#12503=ORIENTED_EDGE('',*,*,#9639,.F.);
#12504=ORIENTED_EDGE('',*,*,#9640,.F.);
#12505=ORIENTED_EDGE('',*,*,#9637,.T.);
#12506=ORIENTED_EDGE('',*,*,#9638,.T.);
#12507=ORIENTED_EDGE('',*,*,#9640,.T.);
#12508=ORIENTED_EDGE('',*,*,#9617,.F.);
#12509=ORIENTED_EDGE('',*,*,#9613,.F.);
#12510=ORIENTED_EDGE('',*,*,#9622,.T.);
#12511=ORIENTED_EDGE('',*,*,#9641,.T.);
#12512=ORIENTED_EDGE('',*,*,#9621,.T.);
#12513=ORIENTED_EDGE('',*,*,#9642,.T.);
#12514=ORIENTED_EDGE('',*,*,#9628,.T.);
#12515=ORIENTED_EDGE('',*,*,#9643,.T.);
#12516=ORIENTED_EDGE('',*,*,#9627,.T.);
#12517=ORIENTED_EDGE('',*,*,#9644,.T.);
#12518=ORIENTED_EDGE('',*,*,#9626,.T.);
#12519=ORIENTED_EDGE('',*,*,#9645,.T.);
#12520=ORIENTED_EDGE('',*,*,#9625,.T.);
#12521=ORIENTED_EDGE('',*,*,#9646,.T.);
#12522=ORIENTED_EDGE('',*,*,#9624,.T.);
#12523=ORIENTED_EDGE('',*,*,#9647,.T.);
#12524=ORIENTED_EDGE('',*,*,#9623,.T.);
#12525=ORIENTED_EDGE('',*,*,#9648,.T.);
#12526=ORIENTED_EDGE('',*,*,#9649,.T.);
#12527=ORIENTED_EDGE('',*,*,#9650,.T.);
#12528=ORIENTED_EDGE('',*,*,#9651,.F.);
#12529=ORIENTED_EDGE('',*,*,#9652,.F.);
#12530=ORIENTED_EDGE('',*,*,#9653,.T.);
#12531=ORIENTED_EDGE('',*,*,#9652,.T.);
#12532=ORIENTED_EDGE('',*,*,#9654,.F.);
#12533=ORIENTED_EDGE('',*,*,#9650,.F.);
#12534=ORIENTED_EDGE('',*,*,#9655,.F.);
#12535=ORIENTED_EDGE('',*,*,#9656,.T.);
#12536=ORIENTED_EDGE('',*,*,#9657,.F.);
#12537=ORIENTED_EDGE('',*,*,#9658,.F.);
#12538=ORIENTED_EDGE('',*,*,#9659,.F.);
#12539=ORIENTED_EDGE('',*,*,#9660,.F.);
#12540=ORIENTED_EDGE('',*,*,#9661,.F.);
#12541=ORIENTED_EDGE('',*,*,#9662,.F.);
#12542=ORIENTED_EDGE('',*,*,#9663,.F.);
#12543=ORIENTED_EDGE('',*,*,#9664,.F.);
#12544=ORIENTED_EDGE('',*,*,#9656,.F.);
#12545=ORIENTED_EDGE('',*,*,#9665,.F.);
#12546=ORIENTED_EDGE('',*,*,#9666,.F.);
#12547=ORIENTED_EDGE('',*,*,#9667,.T.);
#12548=ORIENTED_EDGE('',*,*,#9668,.F.);
#12549=ORIENTED_EDGE('',*,*,#9669,.F.);
#12550=ORIENTED_EDGE('',*,*,#9667,.F.);
#12551=ORIENTED_EDGE('',*,*,#9670,.F.);
#12552=ORIENTED_EDGE('',*,*,#9654,.T.);
#12553=ORIENTED_EDGE('',*,*,#9651,.T.);
#12554=ORIENTED_EDGE('',*,*,#9671,.F.);
#12555=ORIENTED_EDGE('',*,*,#9665,.T.);
#12556=ORIENTED_EDGE('',*,*,#9672,.F.);
#12557=ORIENTED_EDGE('',*,*,#9673,.F.);
#12558=ORIENTED_EDGE('',*,*,#9674,.F.);
#12559=ORIENTED_EDGE('',*,*,#9655,.T.);
#12560=ORIENTED_EDGE('',*,*,#9673,.T.);
#12561=ORIENTED_EDGE('',*,*,#9675,.F.);
#12562=ORIENTED_EDGE('',*,*,#9676,.F.);
#12563=ORIENTED_EDGE('',*,*,#9677,.T.);
#12564=ORIENTED_EDGE('',*,*,#9674,.T.);
#12565=ORIENTED_EDGE('',*,*,#9677,.F.);
#12566=ORIENTED_EDGE('',*,*,#9678,.F.);
#12567=ORIENTED_EDGE('',*,*,#9675,.T.);
#12568=ORIENTED_EDGE('',*,*,#9676,.T.);
#12569=ORIENTED_EDGE('',*,*,#9678,.T.);
#12570=ORIENTED_EDGE('',*,*,#9653,.F.);
#12571=ORIENTED_EDGE('',*,*,#9649,.F.);
#12572=ORIENTED_EDGE('',*,*,#9661,.T.);
#12573=ORIENTED_EDGE('',*,*,#9679,.F.);
#12574=ORIENTED_EDGE('',*,*,#9660,.T.);
#12575=ORIENTED_EDGE('',*,*,#9680,.F.);
#12576=ORIENTED_EDGE('',*,*,#9659,.T.);
#12577=ORIENTED_EDGE('',*,*,#9681,.F.);
#12578=ORIENTED_EDGE('',*,*,#9658,.T.);
#12579=ORIENTED_EDGE('',*,*,#9682,.F.);
#12580=ORIENTED_EDGE('',*,*,#9657,.T.);
#12581=ORIENTED_EDGE('',*,*,#9683,.F.);
#12582=ORIENTED_EDGE('',*,*,#9664,.T.);
#12583=ORIENTED_EDGE('',*,*,#9684,.F.);
#12584=ORIENTED_EDGE('',*,*,#9663,.T.);
#12585=ORIENTED_EDGE('',*,*,#9685,.F.);
#12586=ORIENTED_EDGE('',*,*,#9662,.T.);
#12587=ORIENTED_EDGE('',*,*,#9686,.F.);
#12588=ORIENTED_EDGE('',*,*,#9646,.F.);
#12589=ORIENTED_EDGE('',*,*,#9687,.T.);
#12590=ORIENTED_EDGE('',*,*,#9688,.T.);
#12591=ORIENTED_EDGE('',*,*,#9689,.F.);
#12592=ORIENTED_EDGE('',*,*,#9643,.F.);
#12593=ORIENTED_EDGE('',*,*,#9644,.F.);
#12594=ORIENTED_EDGE('',*,*,#9645,.F.);
#12595=ORIENTED_EDGE('',*,*,#9690,.F.);
#12596=ORIENTED_EDGE('',*,*,#9691,.F.);
#12597=ORIENTED_EDGE('',*,*,#9692,.F.);
#12598=ORIENTED_EDGE('',*,*,#9693,.F.);
#12599=ORIENTED_EDGE('',*,*,#9694,.F.);
#12600=ORIENTED_EDGE('',*,*,#9695,.F.);
#12601=ORIENTED_EDGE('',*,*,#9696,.F.);
#12602=ORIENTED_EDGE('',*,*,#9697,.F.);
#12603=ORIENTED_EDGE('',*,*,#9680,.T.);
#12604=ORIENTED_EDGE('',*,*,#9681,.T.);
#12605=ORIENTED_EDGE('',*,*,#9682,.T.);
#12606=ORIENTED_EDGE('',*,*,#9683,.T.);
#12607=ORIENTED_EDGE('',*,*,#9698,.T.);
#12608=ORIENTED_EDGE('',*,*,#9699,.F.);
#12609=ORIENTED_EDGE('',*,*,#9700,.F.);
#12610=ORIENTED_EDGE('',*,*,#9701,.F.);
#12611=ORIENTED_EDGE('',*,*,#9702,.T.);
#12612=ORIENTED_EDGE('',*,*,#9703,.T.);
#12613=ORIENTED_EDGE('',*,*,#9704,.F.);
#12614=ORIENTED_EDGE('',*,*,#9705,.T.);
#12615=ORIENTED_EDGE('',*,*,#9706,.T.);
#12616=ORIENTED_EDGE('',*,*,#9707,.T.);
#12617=ORIENTED_EDGE('',*,*,#9708,.T.);
#12618=ORIENTED_EDGE('',*,*,#9709,.T.);
#12619=ORIENTED_EDGE('',*,*,#9710,.T.);
#12620=ORIENTED_EDGE('',*,*,#9711,.F.);
#12621=ORIENTED_EDGE('',*,*,#9712,.F.);
#12622=ORIENTED_EDGE('',*,*,#9713,.T.);
#12623=ORIENTED_EDGE('',*,*,#9714,.T.);
#12624=ORIENTED_EDGE('',*,*,#9672,.T.);
#12625=ORIENTED_EDGE('',*,*,#9668,.T.);
#12626=ORIENTED_EDGE('',*,*,#9669,.T.);
#12627=ORIENTED_EDGE('',*,*,#9715,.T.);
#12628=ORIENTED_EDGE('',*,*,#9716,.F.);
#12629=ORIENTED_EDGE('',*,*,#9715,.F.);
#12630=ORIENTED_EDGE('',*,*,#9670,.T.);
#12631=ORIENTED_EDGE('',*,*,#9666,.T.);
#12632=ORIENTED_EDGE('',*,*,#9671,.T.);
#12633=ORIENTED_EDGE('',*,*,#9714,.F.);
#12634=ORIENTED_EDGE('',*,*,#9632,.T.);
#12635=ORIENTED_EDGE('',*,*,#9633,.T.);
#12636=ORIENTED_EDGE('',*,*,#9630,.T.);
#12637=ORIENTED_EDGE('',*,*,#9634,.T.);
#12638=ORIENTED_EDGE('',*,*,#9717,.T.);
#12639=ORIENTED_EDGE('',*,*,#9718,.T.);
#12640=ORIENTED_EDGE('',*,*,#9699,.T.);
#12641=ORIENTED_EDGE('',*,*,#9719,.T.);
#12642=ORIENTED_EDGE('',*,*,#9720,.T.);
#12643=ORIENTED_EDGE('',*,*,#9721,.F.);
#12644=ORIENTED_EDGE('',*,*,#9720,.F.);
#12645=ORIENTED_EDGE('',*,*,#9722,.T.);
#12646=ORIENTED_EDGE('',*,*,#9718,.F.);
#12647=ORIENTED_EDGE('',*,*,#9688,.F.);
#12648=ORIENTED_EDGE('',*,*,#9723,.F.);
#12649=ORIENTED_EDGE('',*,*,#9724,.T.);
#12650=ORIENTED_EDGE('',*,*,#9693,.T.);
#12651=ORIENTED_EDGE('',*,*,#9725,.F.);
#12652=ORIENTED_EDGE('',*,*,#9726,.F.);
#12653=ORIENTED_EDGE('',*,*,#9727,.T.);
#12654=ORIENTED_EDGE('',*,*,#9728,.T.);
#12655=ORIENTED_EDGE('',*,*,#9704,.T.);
#12656=ORIENTED_EDGE('',*,*,#9729,.F.);
#12657=ORIENTED_EDGE('',*,*,#9730,.T.);
#12658=ORIENTED_EDGE('',*,*,#9731,.T.);
#12659=ORIENTED_EDGE('',*,*,#9732,.F.);
#12660=ORIENTED_EDGE('',*,*,#9702,.F.);
#12661=ORIENTED_EDGE('',*,*,#9695,.T.);
#12662=ORIENTED_EDGE('',*,*,#9733,.T.);
#12663=ORIENTED_EDGE('',*,*,#9734,.T.);
#12664=ORIENTED_EDGE('',*,*,#9735,.F.);
#12665=ORIENTED_EDGE('',*,*,#9703,.F.);
#12666=ORIENTED_EDGE('',*,*,#9732,.T.);
#12667=ORIENTED_EDGE('',*,*,#9736,.T.);
#12668=ORIENTED_EDGE('',*,*,#9737,.T.);
#12669=ORIENTED_EDGE('',*,*,#9738,.T.);
#12670=ORIENTED_EDGE('',*,*,#9739,.F.);
#12671=ORIENTED_EDGE('',*,*,#9696,.T.);
#12672=ORIENTED_EDGE('',*,*,#9735,.T.);
#12673=ORIENTED_EDGE('',*,*,#9740,.F.);
#12674=ORIENTED_EDGE('',*,*,#9725,.T.);
#12675=ORIENTED_EDGE('',*,*,#9692,.T.);
#12676=ORIENTED_EDGE('',*,*,#9741,.T.);
#12677=ORIENTED_EDGE('',*,*,#9742,.T.);
#12678=ORIENTED_EDGE('',*,*,#9743,.F.);
#12679=ORIENTED_EDGE('',*,*,#9744,.T.);
#12680=ORIENTED_EDGE('',*,*,#9729,.T.);
#12681=ORIENTED_EDGE('',*,*,#9745,.F.);
#12682=ORIENTED_EDGE('',*,*,#9746,.F.);
#12683=ORIENTED_EDGE('',*,*,#9747,.F.);
#12684=ORIENTED_EDGE('',*,*,#9748,.T.);
#12685=ORIENTED_EDGE('',*,*,#9749,.F.);
#12686=ORIENTED_EDGE('',*,*,#9750,.F.);
#12687=ORIENTED_EDGE('',*,*,#9709,.F.);
#12688=ORIENTED_EDGE('',*,*,#9751,.T.);
#12689=ORIENTED_EDGE('',*,*,#9752,.F.);
#12690=ORIENTED_EDGE('',*,*,#9753,.F.);
#12691=ORIENTED_EDGE('',*,*,#9754,.F.);
#12692=ORIENTED_EDGE('',*,*,#9755,.T.);
#12693=ORIENTED_EDGE('',*,*,#9756,.F.);
#12694=ORIENTED_EDGE('',*,*,#9757,.F.);
#12695=ORIENTED_EDGE('',*,*,#9758,.F.);
#12696=ORIENTED_EDGE('',*,*,#9759,.T.);
#12697=ORIENTED_EDGE('',*,*,#9760,.F.);
#12698=ORIENTED_EDGE('',*,*,#9761,.F.);
#12699=ORIENTED_EDGE('',*,*,#9762,.F.);
#12700=ORIENTED_EDGE('',*,*,#9763,.T.);
#12701=ORIENTED_EDGE('',*,*,#9764,.F.);
#12702=ORIENTED_EDGE('',*,*,#9765,.F.);
#12703=ORIENTED_EDGE('',*,*,#9766,.T.);
#12704=ORIENTED_EDGE('',*,*,#9767,.F.);
#12705=ORIENTED_EDGE('',*,*,#9768,.T.);
#12706=ORIENTED_EDGE('',*,*,#9769,.T.);
#12707=ORIENTED_EDGE('',*,*,#9770,.F.);
#12708=ORIENTED_EDGE('',*,*,#9771,.F.);
#12709=ORIENTED_EDGE('',*,*,#9772,.T.);
#12710=ORIENTED_EDGE('',*,*,#9773,.F.);
#12711=ORIENTED_EDGE('',*,*,#9774,.T.);
#12712=ORIENTED_EDGE('',*,*,#9775,.F.);
#12713=ORIENTED_EDGE('',*,*,#9776,.F.);
#12714=ORIENTED_EDGE('',*,*,#9777,.F.);
#12715=ORIENTED_EDGE('',*,*,#9778,.T.);
#12716=ORIENTED_EDGE('',*,*,#9779,.F.);
#12717=ORIENTED_EDGE('',*,*,#9780,.F.);
#12718=ORIENTED_EDGE('',*,*,#9781,.F.);
#12719=ORIENTED_EDGE('',*,*,#9782,.T.);
#12720=ORIENTED_EDGE('',*,*,#9747,.T.);
#12721=ORIENTED_EDGE('',*,*,#9783,.T.);
#12722=ORIENTED_EDGE('',*,*,#9784,.F.);
#12723=ORIENTED_EDGE('',*,*,#9785,.F.);
#12724=ORIENTED_EDGE('',*,*,#9754,.T.);
#12725=ORIENTED_EDGE('',*,*,#9786,.T.);
#12726=ORIENTED_EDGE('',*,*,#9787,.F.);
#12727=ORIENTED_EDGE('',*,*,#9788,.F.);
#12728=ORIENTED_EDGE('',*,*,#9758,.T.);
#12729=ORIENTED_EDGE('',*,*,#9789,.T.);
#12730=ORIENTED_EDGE('',*,*,#9790,.F.);
#12731=ORIENTED_EDGE('',*,*,#9791,.F.);
#12732=ORIENTED_EDGE('',*,*,#9762,.T.);
#12733=ORIENTED_EDGE('',*,*,#9792,.T.);
#12734=ORIENTED_EDGE('',*,*,#9793,.F.);
#12735=ORIENTED_EDGE('',*,*,#9794,.F.);
#12736=ORIENTED_EDGE('',*,*,#9767,.T.);
#12737=ORIENTED_EDGE('',*,*,#9795,.T.);
#12738=ORIENTED_EDGE('',*,*,#9796,.F.);
#12739=ORIENTED_EDGE('',*,*,#9797,.T.);
#12740=ORIENTED_EDGE('',*,*,#9798,.F.);
#12741=ORIENTED_EDGE('',*,*,#9781,.T.);
#12742=ORIENTED_EDGE('',*,*,#9799,.T.);
#12743=ORIENTED_EDGE('',*,*,#9800,.F.);
#12744=ORIENTED_EDGE('',*,*,#9773,.T.);
#12745=ORIENTED_EDGE('',*,*,#9801,.T.);
#12746=ORIENTED_EDGE('',*,*,#9802,.F.);
#12747=ORIENTED_EDGE('',*,*,#9803,.F.);
#12748=ORIENTED_EDGE('',*,*,#9777,.T.);
#12749=ORIENTED_EDGE('',*,*,#9804,.T.);
#12750=ORIENTED_EDGE('',*,*,#9805,.F.);
#12751=ORIENTED_EDGE('',*,*,#9806,.F.);
#12752=ORIENTED_EDGE('',*,*,#9716,.T.);
#12753=ORIENTED_EDGE('',*,*,#9717,.F.);
#12754=ORIENTED_EDGE('',*,*,#9713,.F.);
#12755=ORIENTED_EDGE('',*,*,#9721,.T.);
#12756=ORIENTED_EDGE('',*,*,#9737,.F.);
#12757=ORIENTED_EDGE('',*,*,#9807,.T.);
#12758=ORIENTED_EDGE('',*,*,#9808,.T.);
#12759=ORIENTED_EDGE('',*,*,#9809,.F.);
#12760=ORIENTED_EDGE('',*,*,#9810,.T.);
#12761=ORIENTED_EDGE('',*,*,#9811,.F.);
#12762=ORIENTED_EDGE('',*,*,#9738,.F.);
#12763=ORIENTED_EDGE('',*,*,#9809,.T.);
#12764=ORIENTED_EDGE('',*,*,#9812,.F.);
#12765=ORIENTED_EDGE('',*,*,#9697,.T.);
#12766=ORIENTED_EDGE('',*,*,#9739,.T.);
#12767=ORIENTED_EDGE('',*,*,#9811,.T.);
#12768=ORIENTED_EDGE('',*,*,#9741,.F.);
#12769=ORIENTED_EDGE('',*,*,#9691,.T.);
#12770=ORIENTED_EDGE('',*,*,#9813,.T.);
#12771=ORIENTED_EDGE('',*,*,#9814,.F.);
#12772=ORIENTED_EDGE('',*,*,#9815,.T.);
#12773=ORIENTED_EDGE('',*,*,#9816,.F.);
#12774=ORIENTED_EDGE('',*,*,#9742,.F.);
#12775=ORIENTED_EDGE('',*,*,#9814,.T.);
#12776=ORIENTED_EDGE('',*,*,#9817,.F.);
#12777=ORIENTED_EDGE('',*,*,#9818,.T.);
#12778=ORIENTED_EDGE('',*,*,#9743,.T.);
#12779=ORIENTED_EDGE('',*,*,#9816,.T.);
#12780=ORIENTED_EDGE('',*,*,#9730,.F.);
#12781=ORIENTED_EDGE('',*,*,#9701,.T.);
#12782=ORIENTED_EDGE('',*,*,#9728,.F.);
#12783=ORIENTED_EDGE('',*,*,#9819,.T.);
#12784=ORIENTED_EDGE('',*,*,#9817,.T.);
#12785=ORIENTED_EDGE('',*,*,#9815,.F.);
#12786=ORIENTED_EDGE('',*,*,#9813,.F.);
#12787=ORIENTED_EDGE('',*,*,#9690,.T.);
#12788=ORIENTED_EDGE('',*,*,#9724,.F.);
#12789=ORIENTED_EDGE('',*,*,#9820,.T.);
#12790=ORIENTED_EDGE('',*,*,#9733,.F.);
#12791=ORIENTED_EDGE('',*,*,#9694,.T.);
#12792=ORIENTED_EDGE('',*,*,#9812,.T.);
#12793=ORIENTED_EDGE('',*,*,#9810,.F.);
#12794=ORIENTED_EDGE('',*,*,#9808,.F.);
#12795=ORIENTED_EDGE('',*,*,#9821,.T.);
#12796=ORIENTED_EDGE('',*,*,#9705,.F.);
#12797=ORIENTED_EDGE('',*,*,#9822,.T.);
#12798=ORIENTED_EDGE('',*,*,#9823,.T.);
#12799=ORIENTED_EDGE('',*,*,#9824,.T.);
#12800=ORIENTED_EDGE('',*,*,#9784,.T.);
#12801=ORIENTED_EDGE('',*,*,#9825,.F.);
#12802=ORIENTED_EDGE('',*,*,#9826,.T.);
#12803=ORIENTED_EDGE('',*,*,#9827,.T.);
#12804=ORIENTED_EDGE('',*,*,#9800,.T.);
#12805=ORIENTED_EDGE('',*,*,#9828,.F.);
#12806=ORIENTED_EDGE('',*,*,#9829,.T.);
#12807=ORIENTED_EDGE('',*,*,#9830,.T.);
#12808=ORIENTED_EDGE('',*,*,#9805,.T.);
#12809=ORIENTED_EDGE('',*,*,#9831,.F.);
#12810=ORIENTED_EDGE('',*,*,#9832,.T.);
#12811=ORIENTED_EDGE('',*,*,#9833,.T.);
#12812=ORIENTED_EDGE('',*,*,#9802,.T.);
#12813=ORIENTED_EDGE('',*,*,#9834,.F.);
#12814=ORIENTED_EDGE('',*,*,#9835,.F.);
#12815=ORIENTED_EDGE('',*,*,#9836,.T.);
#12816=ORIENTED_EDGE('',*,*,#9837,.T.);
#12817=ORIENTED_EDGE('',*,*,#9838,.F.);
#12818=ORIENTED_EDGE('',*,*,#9796,.T.);
#12819=ORIENTED_EDGE('',*,*,#9839,.F.);
#12820=ORIENTED_EDGE('',*,*,#9840,.F.);
#12821=ORIENTED_EDGE('',*,*,#9841,.T.);
#12822=ORIENTED_EDGE('',*,*,#9842,.T.);
#12823=ORIENTED_EDGE('',*,*,#9793,.T.);
#12824=ORIENTED_EDGE('',*,*,#9843,.F.);
#12825=ORIENTED_EDGE('',*,*,#9844,.T.);
#12826=ORIENTED_EDGE('',*,*,#9845,.T.);
#12827=ORIENTED_EDGE('',*,*,#9790,.T.);
#12828=ORIENTED_EDGE('',*,*,#9846,.F.);
#12829=ORIENTED_EDGE('',*,*,#9847,.T.);
#12830=ORIENTED_EDGE('',*,*,#9848,.T.);
#12831=ORIENTED_EDGE('',*,*,#9787,.T.);
#12832=ORIENTED_EDGE('',*,*,#9849,.F.);
#12833=ORIENTED_EDGE('',*,*,#9850,.T.);
#12834=ORIENTED_EDGE('',*,*,#9851,.T.);
#12835=ORIENTED_EDGE('',*,*,#9711,.T.);
#12836=ORIENTED_EDGE('',*,*,#9852,.F.);
#12837=ORIENTED_EDGE('',*,*,#9853,.T.);
#12838=ORIENTED_EDGE('',*,*,#9854,.T.);
#12839=ORIENTED_EDGE('',*,*,#9855,.F.);
#12840=ORIENTED_EDGE('',*,*,#9707,.F.);
#12841=ORIENTED_EDGE('',*,*,#9856,.F.);
#12842=ORIENTED_EDGE('',*,*,#9857,.F.);
#12843=ORIENTED_EDGE('',*,*,#9740,.T.);
#12844=ORIENTED_EDGE('',*,*,#9734,.F.);
#12845=ORIENTED_EDGE('',*,*,#9820,.F.);
#12846=ORIENTED_EDGE('',*,*,#9726,.T.);
#12847=ORIENTED_EDGE('',*,*,#9858,.T.);
#12848=ORIENTED_EDGE('',*,*,#9829,.F.);
#12849=ORIENTED_EDGE('',*,*,#9859,.F.);
#12850=ORIENTED_EDGE('',*,*,#9779,.T.);
#12851=ORIENTED_EDGE('',*,*,#9799,.F.);
#12852=ORIENTED_EDGE('',*,*,#9780,.T.);
#12853=ORIENTED_EDGE('',*,*,#9859,.T.);
#12854=ORIENTED_EDGE('',*,*,#9828,.T.);
#12855=ORIENTED_EDGE('',*,*,#9778,.F.);
#12856=ORIENTED_EDGE('',*,*,#9806,.T.);
#12857=ORIENTED_EDGE('',*,*,#9830,.F.);
#12858=ORIENTED_EDGE('',*,*,#9858,.F.);
#12859=ORIENTED_EDGE('',*,*,#9860,.T.);
#12860=ORIENTED_EDGE('',*,*,#9832,.F.);
#12861=ORIENTED_EDGE('',*,*,#9861,.F.);
#12862=ORIENTED_EDGE('',*,*,#9775,.T.);
#12863=ORIENTED_EDGE('',*,*,#9804,.F.);
#12864=ORIENTED_EDGE('',*,*,#9776,.T.);
#12865=ORIENTED_EDGE('',*,*,#9861,.T.);
#12866=ORIENTED_EDGE('',*,*,#9831,.T.);
#12867=ORIENTED_EDGE('',*,*,#9774,.F.);
#12868=ORIENTED_EDGE('',*,*,#9803,.T.);
#12869=ORIENTED_EDGE('',*,*,#9833,.F.);
#12870=ORIENTED_EDGE('',*,*,#9860,.F.);
#12871=ORIENTED_EDGE('',*,*,#9797,.F.);
#12872=ORIENTED_EDGE('',*,*,#9838,.T.);
#12873=ORIENTED_EDGE('',*,*,#9862,.T.);
#12874=ORIENTED_EDGE('',*,*,#9768,.F.);
#12875=ORIENTED_EDGE('',*,*,#9801,.F.);
#12876=ORIENTED_EDGE('',*,*,#9772,.F.);
#12877=ORIENTED_EDGE('',*,*,#9863,.F.);
#12878=ORIENTED_EDGE('',*,*,#9834,.T.);
#12879=ORIENTED_EDGE('',*,*,#9864,.T.);
#12880=ORIENTED_EDGE('',*,*,#9836,.F.);
#12881=ORIENTED_EDGE('',*,*,#9865,.F.);
#12882=ORIENTED_EDGE('',*,*,#9770,.T.);
#12883=ORIENTED_EDGE('',*,*,#9863,.T.);
#12884=ORIENTED_EDGE('',*,*,#9771,.T.);
#12885=ORIENTED_EDGE('',*,*,#9865,.T.);
#12886=ORIENTED_EDGE('',*,*,#9835,.T.);
#12887=ORIENTED_EDGE('',*,*,#9862,.F.);
#12888=ORIENTED_EDGE('',*,*,#9837,.F.);
#12889=ORIENTED_EDGE('',*,*,#9864,.F.);
#12890=ORIENTED_EDGE('',*,*,#9769,.F.);
#12891=ORIENTED_EDGE('',*,*,#9795,.F.);
#12892=ORIENTED_EDGE('',*,*,#9766,.F.);
#12893=ORIENTED_EDGE('',*,*,#9866,.F.);
#12894=ORIENTED_EDGE('',*,*,#9839,.T.);
#12895=ORIENTED_EDGE('',*,*,#9867,.T.);
#12896=ORIENTED_EDGE('',*,*,#9841,.F.);
#12897=ORIENTED_EDGE('',*,*,#9868,.F.);
#12898=ORIENTED_EDGE('',*,*,#9764,.T.);
#12899=ORIENTED_EDGE('',*,*,#9866,.T.);
#12900=ORIENTED_EDGE('',*,*,#9765,.T.);
#12901=ORIENTED_EDGE('',*,*,#9868,.T.);
#12902=ORIENTED_EDGE('',*,*,#9840,.T.);
#12903=ORIENTED_EDGE('',*,*,#9763,.F.);
#12904=ORIENTED_EDGE('',*,*,#9794,.T.);
#12905=ORIENTED_EDGE('',*,*,#9842,.F.);
#12906=ORIENTED_EDGE('',*,*,#9867,.F.);
#12907=ORIENTED_EDGE('',*,*,#9869,.T.);
#12908=ORIENTED_EDGE('',*,*,#9844,.F.);
#12909=ORIENTED_EDGE('',*,*,#9870,.F.);
#12910=ORIENTED_EDGE('',*,*,#9760,.T.);
#12911=ORIENTED_EDGE('',*,*,#9792,.F.);
#12912=ORIENTED_EDGE('',*,*,#9761,.T.);
#12913=ORIENTED_EDGE('',*,*,#9870,.T.);
#12914=ORIENTED_EDGE('',*,*,#9843,.T.);
#12915=ORIENTED_EDGE('',*,*,#9759,.F.);
#12916=ORIENTED_EDGE('',*,*,#9791,.T.);
#12917=ORIENTED_EDGE('',*,*,#9845,.F.);
#12918=ORIENTED_EDGE('',*,*,#9869,.F.);
#12919=ORIENTED_EDGE('',*,*,#9871,.T.);
#12920=ORIENTED_EDGE('',*,*,#9847,.F.);
#12921=ORIENTED_EDGE('',*,*,#9872,.F.);
#12922=ORIENTED_EDGE('',*,*,#9756,.T.);
#12923=ORIENTED_EDGE('',*,*,#9789,.F.);
#12924=ORIENTED_EDGE('',*,*,#9757,.T.);
#12925=ORIENTED_EDGE('',*,*,#9872,.T.);
#12926=ORIENTED_EDGE('',*,*,#9846,.T.);
#12927=ORIENTED_EDGE('',*,*,#9755,.F.);
#12928=ORIENTED_EDGE('',*,*,#9788,.T.);
#12929=ORIENTED_EDGE('',*,*,#9848,.F.);
#12930=ORIENTED_EDGE('',*,*,#9871,.F.);
#12931=ORIENTED_EDGE('',*,*,#9873,.T.);
#12932=ORIENTED_EDGE('',*,*,#9850,.F.);
#12933=ORIENTED_EDGE('',*,*,#9874,.F.);
#12934=ORIENTED_EDGE('',*,*,#9752,.T.);
#12935=ORIENTED_EDGE('',*,*,#9786,.F.);
#12936=ORIENTED_EDGE('',*,*,#9753,.T.);
#12937=ORIENTED_EDGE('',*,*,#9874,.T.);
#12938=ORIENTED_EDGE('',*,*,#9849,.T.);
#12939=ORIENTED_EDGE('',*,*,#9751,.F.);
#12940=ORIENTED_EDGE('',*,*,#9712,.T.);
#12941=ORIENTED_EDGE('',*,*,#9851,.F.);
#12942=ORIENTED_EDGE('',*,*,#9873,.F.);
#12943=ORIENTED_EDGE('',*,*,#9875,.T.);
#12944=ORIENTED_EDGE('',*,*,#9853,.F.);
#12945=ORIENTED_EDGE('',*,*,#9876,.F.);
#12946=ORIENTED_EDGE('',*,*,#9749,.T.);
#12947=ORIENTED_EDGE('',*,*,#9710,.F.);
#12948=ORIENTED_EDGE('',*,*,#9750,.T.);
#12949=ORIENTED_EDGE('',*,*,#9876,.T.);
#12950=ORIENTED_EDGE('',*,*,#9852,.T.);
#12951=ORIENTED_EDGE('',*,*,#9748,.F.);
#12952=ORIENTED_EDGE('',*,*,#9785,.T.);
#12953=ORIENTED_EDGE('',*,*,#9854,.F.);
#12954=ORIENTED_EDGE('',*,*,#9875,.F.);
#12955=ORIENTED_EDGE('',*,*,#9877,.T.);
#12956=ORIENTED_EDGE('',*,*,#9826,.F.);
#12957=ORIENTED_EDGE('',*,*,#9878,.F.);
#12958=ORIENTED_EDGE('',*,*,#9745,.T.);
#12959=ORIENTED_EDGE('',*,*,#9783,.F.);
#12960=ORIENTED_EDGE('',*,*,#9746,.T.);
#12961=ORIENTED_EDGE('',*,*,#9878,.T.);
#12962=ORIENTED_EDGE('',*,*,#9825,.T.);
#12963=ORIENTED_EDGE('',*,*,#9782,.F.);
#12964=ORIENTED_EDGE('',*,*,#9798,.T.);
#12965=ORIENTED_EDGE('',*,*,#9827,.F.);
#12966=ORIENTED_EDGE('',*,*,#9877,.F.);
#12967=ORIENTED_EDGE('',*,*,#9698,.F.);
#12968=ORIENTED_EDGE('',*,*,#9684,.T.);
#12969=ORIENTED_EDGE('',*,*,#9685,.T.);
#12970=ORIENTED_EDGE('',*,*,#9686,.T.);
#12971=ORIENTED_EDGE('',*,*,#9679,.T.);
#12972=ORIENTED_EDGE('',*,*,#9700,.T.);
#12973=ORIENTED_EDGE('',*,*,#9722,.F.);
#12974=ORIENTED_EDGE('',*,*,#9719,.F.);
#12975=ORIENTED_EDGE('',*,*,#9736,.F.);
#12976=ORIENTED_EDGE('',*,*,#9731,.F.);
#12977=ORIENTED_EDGE('',*,*,#9821,.F.);
#12978=ORIENTED_EDGE('',*,*,#9807,.F.);
#12979=ORIENTED_EDGE('',*,*,#9744,.F.);
#12980=ORIENTED_EDGE('',*,*,#9818,.F.);
#12981=ORIENTED_EDGE('',*,*,#9819,.F.);
#12982=ORIENTED_EDGE('',*,*,#9727,.F.);
#12983=ORIENTED_EDGE('',*,*,#9687,.F.);
#12984=ORIENTED_EDGE('',*,*,#9647,.F.);
#12985=ORIENTED_EDGE('',*,*,#9648,.F.);
#12986=ORIENTED_EDGE('',*,*,#9641,.F.);
#12987=ORIENTED_EDGE('',*,*,#9642,.F.);
#12988=ORIENTED_EDGE('',*,*,#9689,.T.);
#12989=ORIENTED_EDGE('',*,*,#9723,.T.);
#12990=ORIENTED_EDGE('',*,*,#9708,.F.);
#12991=ORIENTED_EDGE('',*,*,#9855,.T.);
#12992=ORIENTED_EDGE('',*,*,#9879,.F.);
#12993=ORIENTED_EDGE('',*,*,#9822,.F.);
#12994=ORIENTED_EDGE('',*,*,#9880,.T.);
#12995=ORIENTED_EDGE('',*,*,#9856,.T.);
#12996=ORIENTED_EDGE('',*,*,#9706,.F.);
#12997=ORIENTED_EDGE('',*,*,#9824,.F.);
#12998=ORIENTED_EDGE('',*,*,#9879,.T.);
#12999=ORIENTED_EDGE('',*,*,#9857,.T.);
#13000=ORIENTED_EDGE('',*,*,#9880,.F.);
#13001=ORIENTED_EDGE('',*,*,#9823,.F.);
#17348=ADVANCED_FACE('',(#4908),#4594,.T.);
#17349=ADVANCED_FACE('',(#4909),#4595,.F.);
#17350=ADVANCED_FACE('',(#4910),#4596,.F.);
#17351=ADVANCED_FACE('',(#4911),#4597,.T.);
#17352=ADVANCED_FACE('',(#4912,#935),#341,.F.);
#17353=ADVANCED_FACE('',(#4913,#936),#342,.T.);
#17354=ADVANCED_FACE('',(#4914),#343,.T.);
#17355=ADVANCED_FACE('',(#4915),#4598,.F.);
#17356=ADVANCED_FACE('',(#4916),#4599,.T.);
#17357=ADVANCED_FACE('',(#4917),#344,.T.);
#17358=ADVANCED_FACE('',(#4918),#345,.T.);
#17359=ADVANCED_FACE('',(#4919),#4600,.T.);
#17360=ADVANCED_FACE('',(#4920),#4601,.T.);
#17361=ADVANCED_FACE('',(#4921),#4602,.T.);
#17362=ADVANCED_FACE('',(#4922),#4603,.T.);
#17363=ADVANCED_FACE('',(#4923),#4604,.T.);
#17364=ADVANCED_FACE('',(#4924),#4605,.T.);
#17365=ADVANCED_FACE('',(#4925),#4606,.T.);
#17366=ADVANCED_FACE('',(#4926),#4607,.T.);
#17367=ADVANCED_FACE('',(#4927),#4608,.T.);
#17368=ADVANCED_FACE('',(#4928),#4609,.F.);
#17369=ADVANCED_FACE('',(#4929),#4610,.F.);
#17370=ADVANCED_FACE('',(#4930),#4611,.T.);
#17371=ADVANCED_FACE('',(#4931,#937),#346,.F.);
#17372=ADVANCED_FACE('',(#4932,#938),#347,.T.);
#17373=ADVANCED_FACE('',(#4933),#348,.T.);
#17374=ADVANCED_FACE('',(#4934),#4612,.F.);
#17375=ADVANCED_FACE('',(#4935),#4613,.T.);
#17376=ADVANCED_FACE('',(#4936),#349,.T.);
#17377=ADVANCED_FACE('',(#4937),#350,.T.);
#17378=ADVANCED_FACE('',(#939),#4614,.T.);
#17379=ADVANCED_FACE('',(#940),#4615,.T.);
#17380=ADVANCED_FACE('',(#4938),#4616,.T.);
#17381=ADVANCED_FACE('',(#941),#4617,.T.);
#17382=ADVANCED_FACE('',(#942),#4618,.T.);
#17383=ADVANCED_FACE('',(#4939),#4619,.T.);
#17384=ADVANCED_FACE('',(#4940),#4620,.T.);
#17385=ADVANCED_FACE('',(#4941),#4621,.T.);
#17386=ADVANCED_FACE('',(#4942),#244,.F.);
#17387=ADVANCED_FACE('',(#4943),#4622,.F.);
#17388=ADVANCED_FACE('',(#4944),#4623,.F.);
#17389=ADVANCED_FACE('',(#4945),#245,.T.);
#17390=ADVANCED_FACE('',(#4946),#4624,.F.);
#17391=ADVANCED_FACE('',(#4947),#4625,.F.);
#17392=ADVANCED_FACE('',(#4948),#4626,.T.);
#17393=ADVANCED_FACE('',(#4949,#943),#4627,.T.);
#17394=ADVANCED_FACE('',(#4950,#944,#945,#946,#947,#948),#4628,.F.);
#17395=ADVANCED_FACE('',(#4951,#949),#351,.T.);
#17396=ADVANCED_FACE('',(#4952),#4629,.T.);
#17397=ADVANCED_FACE('',(#4953),#4630,.T.);
#17398=ADVANCED_FACE('',(#4954),#4631,.T.);
#17399=ADVANCED_FACE('',(#4955),#4632,.T.);
#17400=ADVANCED_FACE('',(#4956),#4633,.T.);
#17401=ADVANCED_FACE('',(#4957),#4634,.T.);
#17402=ADVANCED_FACE('',(#4958),#4635,.T.);
#17403=ADVANCED_FACE('',(#4959),#4636,.T.);
#17404=ADVANCED_FACE('',(#4960,#950),#352,.T.);
#17405=ADVANCED_FACE('',(#4961,#951),#353,.F.);
#17406=ADVANCED_FACE('',(#4962),#4637,.F.);
#17407=ADVANCED_FACE('',(#4963),#4638,.T.);
#17408=ADVANCED_FACE('',(#4964),#4639,.F.);
#17409=ADVANCED_FACE('',(#4965),#4640,.F.);
#17410=ADVANCED_FACE('',(#4966),#4641,.T.);
#17411=ADVANCED_FACE('',(#4967),#4642,.F.);
#17412=ADVANCED_FACE('',(#4968,#952),#354,.F.);
#17413=ADVANCED_FACE('',(#4969,#953),#355,.T.);
#17414=ADVANCED_FACE('',(#4970),#4643,.F.);
#17415=ADVANCED_FACE('',(#4971),#356,.F.);
#17416=ADVANCED_FACE('',(#4972),#357,.F.);
#17417=ADVANCED_FACE('',(#4973),#358,.T.);
#17418=ADVANCED_FACE('',(#4974),#359,.F.);
#17419=ADVANCED_FACE('',(#4975),#360,.F.);
#17420=ADVANCED_FACE('',(#4976),#361,.T.);
#17421=ADVANCED_FACE('',(#4977),#362,.F.);
#17422=ADVANCED_FACE('',(#4978),#363,.F.);
#17423=ADVANCED_FACE('',(#4979),#364,.F.);
#17424=ADVANCED_FACE('',(#4980),#365,.F.);
#17425=ADVANCED_FACE('',(#4981),#366,.T.);
#17426=ADVANCED_FACE('',(#4982),#367,.F.);
#17427=ADVANCED_FACE('',(#4983),#368,.F.);
#17428=ADVANCED_FACE('',(#4984),#369,.F.);
#17429=ADVANCED_FACE('',(#4985),#370,.T.);
#17430=ADVANCED_FACE('',(#4986),#371,.F.);
#17431=ADVANCED_FACE('',(#4987),#372,.F.);
#17432=ADVANCED_FACE('',(#4988),#373,.T.);
#17433=ADVANCED_FACE('',(#4989),#374,.F.);
#17434=ADVANCED_FACE('',(#4990),#375,.F.);
#17435=ADVANCED_FACE('',(#4991),#376,.T.);
#17436=ADVANCED_FACE('',(#4992),#377,.F.);
#17437=ADVANCED_FACE('',(#4993),#378,.F.);
#17438=ADVANCED_FACE('',(#4994),#379,.T.);
#17439=ADVANCED_FACE('',(#4995),#380,.F.);
#17440=ADVANCED_FACE('',(#4996),#381,.F.);
#17441=ADVANCED_FACE('',(#4997),#382,.T.);
#17442=ADVANCED_FACE('',(#4998),#383,.F.);
#17443=ADVANCED_FACE('',(#4999),#384,.F.);
#17444=ADVANCED_FACE('',(#5000),#385,.T.);
#17445=ADVANCED_FACE('',(#5001),#246,.T.);
#17446=ADVANCED_FACE('',(#5002),#4644,.F.);
#17447=ADVANCED_FACE('',(#5003),#4645,.F.);
#17448=ADVANCED_FACE('',(#5004),#247,.F.);
#17449=ADVANCED_FACE('',(#5005),#386,.F.);
#17450=ADVANCED_FACE('',(#5006),#387,.F.);
#17451=ADVANCED_FACE('',(#5007),#388,.F.);
#18260=CLOSED_SHELL('',(#17348,#17349,#17350,#17351,#17352,#17353,#17354,
#17355,#17356,#17357,#17358,#17359,#17360,#17361,#17362,#17363,#17364,#17365,
#17366,#17367,#17368,#17369,#17370,#17371,#17372,#17373,#17374,#17375,#17376,
#17377,#17378,#17379,#17380,#17381,#17382,#17383,#17384,#17385,#17386,#17387,
#17388,#17389,#17390,#17391,#17392,#17393,#17394,#17395,#17396,#17397,#17398,
#17399,#17400,#17401,#17402,#17403,#17404,#17405,#17406,#17407,#17408,#17409,
#17410,#17411,#17412,#17413,#17414,#17415,#17416,#17417,#17418,#17419,#17420,
#17421,#17422,#17423,#17424,#17425,#17426,#17427,#17428,#17429,#17430,#17431,
#17432,#17433,#17434,#17435,#17436,#17437,#17438,#17439,#17440,#17441,#17442,
#17443,#17444,#17445,#17446,#17447,#17448,#17449,#17450,#17451));
#18536=AXIS2_PLACEMENT_3D('',#25628,#20511,#20512);
#18537=AXIS2_PLACEMENT_3D('',#25629,#20513,#20514);
#18538=AXIS2_PLACEMENT_3D('',#25632,#20515,#20516);
#18539=AXIS2_PLACEMENT_3D('',#25636,#20518,#20519);
#18540=AXIS2_PLACEMENT_3D('',#25638,#20521,#20522);
#18541=AXIS2_PLACEMENT_3D('',#25639,#20523,#20524);
#18542=AXIS2_PLACEMENT_3D('',#25640,#20525,#20526);
#18543=AXIS2_PLACEMENT_3D('',#25641,#20527,#20528);
#18544=AXIS2_PLACEMENT_3D('',#25643,#20529,#20530);
#18545=AXIS2_PLACEMENT_3D('',#25712,#20532,#20533);
#18546=AXIS2_PLACEMENT_3D('',#25715,#20534,#20535);
#18547=AXIS2_PLACEMENT_3D('',#25719,#20537,#20538);
#18548=AXIS2_PLACEMENT_3D('',#25721,#20540,#20541);
#18549=AXIS2_PLACEMENT_3D('',#25722,#20542,#20543);
#18550=AXIS2_PLACEMENT_3D('',#25723,#20544,#20545);
#18551=AXIS2_PLACEMENT_3D('',#25724,#20546,#20547);
#18552=AXIS2_PLACEMENT_3D('',#25727,#20548,#20549);
#18553=AXIS2_PLACEMENT_3D('',#25728,#20550,#20551);
#18554=AXIS2_PLACEMENT_3D('',#25729,#20552,#20553);
#18555=AXIS2_PLACEMENT_3D('',#25730,#20554,#20555);
#18556=AXIS2_PLACEMENT_3D('',#25734,#20557,#20558);
#18557=AXIS2_PLACEMENT_3D('',#25736,#20560,#20561);
#18558=AXIS2_PLACEMENT_3D('',#25737,#20562,#20563);
#18559=AXIS2_PLACEMENT_3D('',#25738,#20564,#20565);
#18560=AXIS2_PLACEMENT_3D('',#25739,#20566,#20567);
#18561=AXIS2_PLACEMENT_3D('',#25740,#20568,#20569);
#18562=AXIS2_PLACEMENT_3D('',#25799,#20570,#20571);
#18563=AXIS2_PLACEMENT_3D('',#25837,#20572,#20573);
#18564=AXIS2_PLACEMENT_3D('',#25890,#20574,#20575);
#18565=AXIS2_PLACEMENT_3D('',#25943,#20576,#20577);
#18566=AXIS2_PLACEMENT_3D('',#25990,#20578,#20579);
#18567=AXIS2_PLACEMENT_3D('',#26046,#20580,#20581);
#18568=AXIS2_PLACEMENT_3D('',#26093,#20582,#20583);
#18569=AXIS2_PLACEMENT_3D('',#26140,#20584,#20585);
#18570=AXIS2_PLACEMENT_3D('',#26143,#20586,#20587);
#18571=AXIS2_PLACEMENT_3D('',#26147,#20589,#20590);
#18572=AXIS2_PLACEMENT_3D('',#26149,#20592,#20593);
#18573=AXIS2_PLACEMENT_3D('',#26150,#20594,#20595);
#18574=AXIS2_PLACEMENT_3D('',#26151,#20596,#20597);
#18575=AXIS2_PLACEMENT_3D('',#26152,#20598,#20599);
#18576=AXIS2_PLACEMENT_3D('',#26154,#20600,#20601);
#18577=AXIS2_PLACEMENT_3D('',#26223,#20603,#20604);
#18578=AXIS2_PLACEMENT_3D('',#26226,#20605,#20606);
#18579=AXIS2_PLACEMENT_3D('',#26230,#20608,#20609);
#18580=AXIS2_PLACEMENT_3D('',#26232,#20611,#20612);
#18581=AXIS2_PLACEMENT_3D('',#26234,#20613,#20614);
#18582=AXIS2_PLACEMENT_3D('',#26235,#20615,#20616);
#18583=AXIS2_PLACEMENT_3D('',#26236,#20617,#20618);
#18584=AXIS2_PLACEMENT_3D('',#26238,#20619,#20620);
#18585=AXIS2_PLACEMENT_3D('',#26239,#20621,#20622);
#18586=AXIS2_PLACEMENT_3D('',#26242,#20623,#20624);
#18587=AXIS2_PLACEMENT_3D('',#26243,#20625,#20626);
#18588=AXIS2_PLACEMENT_3D('',#26244,#20627,#20628);
#18589=AXIS2_PLACEMENT_3D('',#26245,#20629,#20630);
#18590=AXIS2_PLACEMENT_3D('',#26249,#20632,#20633);
#18591=AXIS2_PLACEMENT_3D('',#26251,#20635,#20636);
#18592=AXIS2_PLACEMENT_3D('',#26252,#20637,#20638);
#18593=AXIS2_PLACEMENT_3D('',#26253,#20639,#20640);
#18594=AXIS2_PLACEMENT_3D('',#26254,#20641,#20642);
#18595=AXIS2_PLACEMENT_3D('',#26255,#20643,#20644);
#18596=AXIS2_PLACEMENT_3D('',#26260,#20645,#20646);
#18597=AXIS2_PLACEMENT_3D('',#26265,#20647,#20648);
#18598=AXIS2_PLACEMENT_3D('',#26270,#20649,#20650);
#18599=AXIS2_PLACEMENT_3D('',#26275,#20651,#20652);
#18600=AXIS2_PLACEMENT_3D('',#26282,#20653,#20654);
#18601=AXIS2_PLACEMENT_3D('',#26287,#20655,#20656);
#18602=AXIS2_PLACEMENT_3D('',#26292,#20657,#20658);
#18603=AXIS2_PLACEMENT_3D('',#26345,#20661,#20662);
#18604=AXIS2_PLACEMENT_3D('',#26348,#20663,#20664);
#18605=AXIS2_PLACEMENT_3D('',#26352,#20666,#20667);
#18606=AXIS2_PLACEMENT_3D('',#26354,#20669,#20670);
#18607=AXIS2_PLACEMENT_3D('',#26357,#20671,#20672);
#18608=AXIS2_PLACEMENT_3D('',#26361,#20674,#20675);
#18609=AXIS2_PLACEMENT_3D('',#26563,#20679,#20680);
#18610=AXIS2_PLACEMENT_3D('',#26566,#20681,#20682);
#18611=AXIS2_PLACEMENT_3D('',#26570,#20684,#20685);
#18612=AXIS2_PLACEMENT_3D('',#26572,#20687,#20688);
#18613=AXIS2_PLACEMENT_3D('',#26575,#20689,#20690);
#18614=AXIS2_PLACEMENT_3D('',#26579,#20692,#20693);
#18615=AXIS2_PLACEMENT_3D('',#26581,#20695,#20696);
#18616=AXIS2_PLACEMENT_3D('',#26584,#20697,#20698);
#18617=AXIS2_PLACEMENT_3D('',#26588,#20700,#20701);
#18618=AXIS2_PLACEMENT_3D('',#26590,#20703,#20704);
#18619=AXIS2_PLACEMENT_3D('',#26592,#20705,#20706);
#18620=AXIS2_PLACEMENT_3D('',#26596,#20709,#20710);
#18621=AXIS2_PLACEMENT_3D('',#26597,#20711,#20712);
#18622=AXIS2_PLACEMENT_3D('',#26599,#20713,#20714);
#18623=AXIS2_PLACEMENT_3D('',#26608,#20717,#20718);
#18624=AXIS2_PLACEMENT_3D('',#26806,#20719,#20720);
#18625=AXIS2_PLACEMENT_3D('',#26808,#20721,#20722);
#18626=AXIS2_PLACEMENT_3D('',#26813,#20725,#20726);
#18627=AXIS2_PLACEMENT_3D('',#26814,#20727,#20728);
#18628=AXIS2_PLACEMENT_3D('',#26816,#20729,#20730);
#18629=AXIS2_PLACEMENT_3D('',#26819,#20732,#20733);
#18630=AXIS2_PLACEMENT_3D('',#26821,#20734,#20735);
#18631=AXIS2_PLACEMENT_3D('',#26824,#20737,#20738);
#18632=AXIS2_PLACEMENT_3D('',#26825,#20739,#20740);
#18633=AXIS2_PLACEMENT_3D('',#26827,#20741,#20742);
#18634=AXIS2_PLACEMENT_3D('',#26829,#20743,#20744);
#18635=AXIS2_PLACEMENT_3D('',#26831,#20745,#20746);
#18636=AXIS2_PLACEMENT_3D('',#26832,#20747,#20748);
#18637=AXIS2_PLACEMENT_3D('',#26833,#20749,#20750);
#18638=AXIS2_PLACEMENT_3D('',#26835,#20751,#20752);
#18639=AXIS2_PLACEMENT_3D('',#26837,#20753,#20754);
#18640=AXIS2_PLACEMENT_3D('',#26839,#20755,#20756);
#18641=AXIS2_PLACEMENT_3D('',#26840,#20757,#20758);
#18642=AXIS2_PLACEMENT_3D('',#26847,#20761,#20762);
#18643=AXIS2_PLACEMENT_3D('',#26860,#20769,#20770);
#18644=AXIS2_PLACEMENT_3D('',#26868,#20774,#20775);
#18645=AXIS2_PLACEMENT_3D('',#26876,#20779,#20780);
#18646=AXIS2_PLACEMENT_3D('',#26886,#20785,#20786);
#18647=AXIS2_PLACEMENT_3D('',#26898,#20792,#20793);
#18648=AXIS2_PLACEMENT_3D('',#26906,#20797,#20798);
#18649=AXIS2_PLACEMENT_3D('',#26914,#20802,#20803);
#18650=AXIS2_PLACEMENT_3D('',#26916,#20805,#20806);
#18651=AXIS2_PLACEMENT_3D('',#26920,#20808,#20809);
#18652=AXIS2_PLACEMENT_3D('',#26922,#20811,#20812);
#18653=AXIS2_PLACEMENT_3D('',#26926,#20814,#20815);
#18654=AXIS2_PLACEMENT_3D('',#26928,#20817,#20818);
#18655=AXIS2_PLACEMENT_3D('',#26932,#20820,#20821);
#18656=AXIS2_PLACEMENT_3D('',#26934,#20823,#20824);
#18657=AXIS2_PLACEMENT_3D('',#26938,#20826,#20827);
#18658=AXIS2_PLACEMENT_3D('',#26940,#20829,#20830);
#18659=AXIS2_PLACEMENT_3D('',#26944,#20832,#20833);
#18660=AXIS2_PLACEMENT_3D('',#26946,#20835,#20836);
#18661=AXIS2_PLACEMENT_3D('',#26951,#20839,#20840);
#18662=AXIS2_PLACEMENT_3D('',#26952,#20841,#20842);
#18663=AXIS2_PLACEMENT_3D('',#26956,#20844,#20845);
#18664=AXIS2_PLACEMENT_3D('',#26958,#20847,#20848);
#18665=AXIS2_PLACEMENT_3D('',#26962,#20850,#20851);
#18666=AXIS2_PLACEMENT_3D('',#26964,#20853,#20854);
#18667=AXIS2_PLACEMENT_3D('',#26965,#20855,#20856);
#18668=AXIS2_PLACEMENT_3D('',#26966,#20857,#20858);
#18669=AXIS2_PLACEMENT_3D('',#26970,#20860,#20861);
#18670=AXIS2_PLACEMENT_3D('',#26972,#20863,#20864);
#18671=AXIS2_PLACEMENT_3D('',#26974,#20865,#20866);
#18672=AXIS2_PLACEMENT_3D('',#26976,#20868,#20869);
#18673=AXIS2_PLACEMENT_3D('',#26977,#20870,#20871);
#18674=AXIS2_PLACEMENT_3D('',#26978,#20872,#20873);
#18675=AXIS2_PLACEMENT_3D('',#26980,#20874,#20875);
#18676=AXIS2_PLACEMENT_3D('',#26982,#20877,#20878);
#18677=AXIS2_PLACEMENT_3D('',#26984,#20879,#20880);
#18678=AXIS2_PLACEMENT_3D('',#26986,#20882,#20883);
#18679=AXIS2_PLACEMENT_3D('',#26988,#20884,#20885);
#18680=AXIS2_PLACEMENT_3D('',#26990,#20887,#20888);
#18681=AXIS2_PLACEMENT_3D('',#26991,#20889,#20890);
#18682=AXIS2_PLACEMENT_3D('',#26992,#20891,#20892);
#18683=AXIS2_PLACEMENT_3D('',#26993,#20893,#20894);
#18684=AXIS2_PLACEMENT_3D('',#26999,#20898,#20899);
#18685=AXIS2_PLACEMENT_3D('',#27056,#20933,#20934);
#18686=AXIS2_PLACEMENT_3D('',#27057,#20935,#20936);
#18687=AXIS2_PLACEMENT_3D('',#27060,#20939,#20940);
#18688=AXIS2_PLACEMENT_3D('',#27061,#20941,#20942);
#18689=AXIS2_PLACEMENT_3D('',#27062,#20943,#20944);
#18690=AXIS2_PLACEMENT_3D('',#27065,#20947,#20948);
#18691=AXIS2_PLACEMENT_3D('',#27066,#20949,#20950);
#18692=AXIS2_PLACEMENT_3D('',#27067,#20951,#20952);
#18693=AXIS2_PLACEMENT_3D('',#27069,#20954,#20955);
#18694=AXIS2_PLACEMENT_3D('',#27071,#20957,#20958);
#18695=AXIS2_PLACEMENT_3D('',#27074,#20961,#20962);
#18696=AXIS2_PLACEMENT_3D('',#27075,#20963,#20964);
#18697=AXIS2_PLACEMENT_3D('',#27076,#20965,#20966);
#18698=AXIS2_PLACEMENT_3D('',#27078,#20968,#20969);
#18699=AXIS2_PLACEMENT_3D('',#27081,#20972,#20973);
#18700=AXIS2_PLACEMENT_3D('',#27082,#20974,#20975);
#18701=AXIS2_PLACEMENT_3D('',#27083,#20976,#20977);
#18702=AXIS2_PLACEMENT_3D('',#27086,#20980,#20981);
#18703=AXIS2_PLACEMENT_3D('',#27087,#20982,#20983);
#18704=AXIS2_PLACEMENT_3D('',#27088,#20984,#20985);
#18705=AXIS2_PLACEMENT_3D('',#27091,#20988,#20989);
#18706=AXIS2_PLACEMENT_3D('',#27092,#20990,#20991);
#18707=AXIS2_PLACEMENT_3D('',#27093,#20992,#20993);
#18708=AXIS2_PLACEMENT_3D('',#27096,#20996,#20997);
#18709=AXIS2_PLACEMENT_3D('',#27097,#20998,#20999);
#18710=AXIS2_PLACEMENT_3D('',#27098,#21000,#21001);
#18711=AXIS2_PLACEMENT_3D('',#27101,#21004,#21005);
#18712=AXIS2_PLACEMENT_3D('',#27102,#21006,#21007);
#18713=AXIS2_PLACEMENT_3D('',#27103,#21008,#21009);
#18714=AXIS2_PLACEMENT_3D('',#27106,#21012,#21013);
#18715=AXIS2_PLACEMENT_3D('',#27107,#21014,#21015);
#18716=AXIS2_PLACEMENT_3D('',#27128,#21016,#21017);
#18717=AXIS2_PLACEMENT_3D('',#27129,#21018,#21019);
#18718=AXIS2_PLACEMENT_3D('',#27154,#21020,#21021);
#18719=AXIS2_PLACEMENT_3D('',#27156,#21023,#21024);
#18720=AXIS2_PLACEMENT_3D('',#27158,#21026,#21027);
#20511=DIRECTION('axis',(0.,0.,1.));
#20512=DIRECTION('refdir',(1.,0.,0.));
#20513=DIRECTION('center_axis',(0.,0.,-1.));
#20514=DIRECTION('ref_axis',(-1.,0.,0.));
#20515=DIRECTION('center_axis',(0.,0.,-1.));
#20516=DIRECTION('ref_axis',(1.,0.,0.));
#20517=DIRECTION('',(0.,0.,-1.));
#20518=DIRECTION('center_axis',(0.,0.,-1.));
#20519=DIRECTION('ref_axis',(1.,0.,0.));
#20520=DIRECTION('',(0.,0.,-1.));
#20521=DIRECTION('center_axis',(0.,0.,-1.));
#20522=DIRECTION('ref_axis',(-1.,0.,0.));
#20523=DIRECTION('center_axis',(0.,0.,1.));
#20524=DIRECTION('ref_axis',(1.,0.,0.));
#20525=DIRECTION('center_axis',(0.,0.,1.));
#20526=DIRECTION('ref_axis',(1.,0.,0.));
#20527=DIRECTION('center_axis',(1.,0.,0.));
#20528=DIRECTION('ref_axis',(0.,0.,-1.));
#20529=DIRECTION('center_axis',(1.,0.,0.));
#20530=DIRECTION('ref_axis',(0.,0.,-1.));
#20531=DIRECTION('',(1.,0.,0.));
#20532=DIRECTION('center_axis',(0.,0.,-1.));
#20533=DIRECTION('ref_axis',(-1.,0.,0.));
#20534=DIRECTION('center_axis',(0.,0.,1.));
#20535=DIRECTION('ref_axis',(1.,0.,0.));
#20536=DIRECTION('',(0.,0.,1.));
#20537=DIRECTION('center_axis',(0.,0.,1.));
#20538=DIRECTION('ref_axis',(1.,0.,0.));
#20539=DIRECTION('',(0.,0.,-1.));
#20540=DIRECTION('center_axis',(0.,0.,1.));
#20541=DIRECTION('ref_axis',(1.,0.,0.));
#20542=DIRECTION('center_axis',(0.,0.,-1.));
#20543=DIRECTION('ref_axis',(-1.,0.,0.));
#20544=DIRECTION('center_axis',(0.,0.,1.));
#20545=DIRECTION('ref_axis',(1.,0.,0.));
#20546=DIRECTION('center_axis',(0.,0.,1.));
#20547=DIRECTION('ref_axis',(-1.,0.,0.));
#20548=DIRECTION('center_axis',(0.,0.,1.));
#20549=DIRECTION('ref_axis',(1.,0.,0.));
#20550=DIRECTION('center_axis',(0.,0.,-1.));
#20551=DIRECTION('ref_axis',(1.,0.,0.));
#20552=DIRECTION('center_axis',(1.,0.,0.));
#20553=DIRECTION('ref_axis',(0.,0.,-1.));
#20554=DIRECTION('center_axis',(0.,0.,1.));
#20555=DIRECTION('ref_axis',(-1.,1.22464679914735E-16,0.));
#20556=DIRECTION('',(0.,0.,1.));
#20557=DIRECTION('center_axis',(0.,0.,1.));
#20558=DIRECTION('ref_axis',(1.,0.,0.));
#20559=DIRECTION('',(0.,0.,1.));
#20560=DIRECTION('center_axis',(0.,0.,1.));
#20561=DIRECTION('ref_axis',(-1.,1.22464679914735E-16,0.));
#20562=DIRECTION('center_axis',(0.,0.,-1.));
#20563=DIRECTION('ref_axis',(1.,0.,0.));
#20564=DIRECTION('center_axis',(0.,0.,1.));
#20565=DIRECTION('ref_axis',(1.,0.,0.));
#20566=DIRECTION('center_axis',(0.,0.,-1.));
#20567=DIRECTION('ref_axis',(1.,0.,0.));
#20568=DIRECTION('center_axis',(0.,0.,-1.));
#20569=DIRECTION('ref_axis',(-1.,0.,0.));
#20570=DIRECTION('center_axis',(0.,0.,-1.));
#20571=DIRECTION('ref_axis',(-1.,0.,0.));
#20572=DIRECTION('center_axis',(0.,0.,-1.));
#20573=DIRECTION('ref_axis',(-1.,0.,0.));
#20574=DIRECTION('center_axis',(0.,0.,-1.));
#20575=DIRECTION('ref_axis',(-1.,0.,0.));
#20576=DIRECTION('center_axis',(0.,0.,-1.));
#20577=DIRECTION('ref_axis',(-1.,0.,0.));
#20578=DIRECTION('center_axis',(0.,0.,-1.));
#20579=DIRECTION('ref_axis',(-1.,0.,0.));
#20580=DIRECTION('center_axis',(0.,0.,-1.));
#20581=DIRECTION('ref_axis',(-1.,0.,0.));
#20582=DIRECTION('center_axis',(0.,0.,-1.));
#20583=DIRECTION('ref_axis',(-1.,0.,0.));
#20584=DIRECTION('center_axis',(0.,0.,1.));
#20585=DIRECTION('ref_axis',(1.,0.,0.));
#20586=DIRECTION('center_axis',(0.,0.,1.));
#20587=DIRECTION('ref_axis',(-1.,0.,0.));
#20588=DIRECTION('',(0.,0.,1.));
#20589=DIRECTION('center_axis',(0.,0.,1.));
#20590=DIRECTION('ref_axis',(-1.,0.,0.));
#20591=DIRECTION('',(0.,0.,1.));
#20592=DIRECTION('center_axis',(0.,0.,1.));
#20593=DIRECTION('ref_axis',(1.,0.,0.));
#20594=DIRECTION('center_axis',(0.,0.,-1.));
#20595=DIRECTION('ref_axis',(-1.,0.,0.));
#20596=DIRECTION('center_axis',(0.,0.,-1.));
#20597=DIRECTION('ref_axis',(-1.,0.,0.));
#20598=DIRECTION('center_axis',(-1.,0.,0.));
#20599=DIRECTION('ref_axis',(0.,0.,1.));
#20600=DIRECTION('center_axis',(-1.,0.,0.));
#20601=DIRECTION('ref_axis',(0.,0.,1.));
#20602=DIRECTION('',(-1.,0.,0.));
#20603=DIRECTION('center_axis',(0.,0.,1.));
#20604=DIRECTION('ref_axis',(1.,0.,0.));
#20605=DIRECTION('center_axis',(0.,0.,-1.));
#20606=DIRECTION('ref_axis',(-1.,0.,0.));
#20607=DIRECTION('',(0.,0.,-1.));
#20608=DIRECTION('center_axis',(0.,0.,-1.));
#20609=DIRECTION('ref_axis',(-1.,0.,0.));
#20610=DIRECTION('',(0.,0.,1.));
#20611=DIRECTION('center_axis',(0.,0.,-1.));
#20612=DIRECTION('ref_axis',(-1.,0.,0.));
#20613=DIRECTION('center_axis',(0.,0.,1.));
#20614=DIRECTION('ref_axis',(-1.,0.,0.));
#20615=DIRECTION('center_axis',(0.,0.,1.));
#20616=DIRECTION('ref_axis',(-1.,0.,0.));
#20617=DIRECTION('center_axis',(0.,0.,-1.));
#20618=DIRECTION('ref_axis',(-1.,0.,0.));
#20619=DIRECTION('center_axis',(0.,0.,-1.));
#20620=DIRECTION('ref_axis',(-1.,0.,0.));
#20621=DIRECTION('center_axis',(0.,0.,-1.));
#20622=DIRECTION('ref_axis',(-1.,0.,0.));
#20623=DIRECTION('center_axis',(0.,0.,-1.));
#20624=DIRECTION('ref_axis',(-1.,0.,0.));
#20625=DIRECTION('center_axis',(0.,0.,1.));
#20626=DIRECTION('ref_axis',(-1.,0.,0.));
#20627=DIRECTION('center_axis',(-1.,0.,0.));
#20628=DIRECTION('ref_axis',(0.,0.,1.));
#20629=DIRECTION('center_axis',(0.,0.,-1.));
#20630=DIRECTION('ref_axis',(1.,1.22464679914735E-16,0.));
#20631=DIRECTION('',(0.,0.,-1.));
#20632=DIRECTION('center_axis',(0.,0.,-1.));
#20633=DIRECTION('ref_axis',(-1.,0.,0.));
#20634=DIRECTION('',(0.,0.,-1.));
#20635=DIRECTION('center_axis',(0.,0.,-1.));
#20636=DIRECTION('ref_axis',(1.,1.22464679914735E-16,0.));
#20637=DIRECTION('center_axis',(0.,0.,1.));
#20638=DIRECTION('ref_axis',(-1.,0.,0.));
#20639=DIRECTION('center_axis',(0.,0.,-1.));
#20640=DIRECTION('ref_axis',(-1.,0.,0.));
#20641=DIRECTION('center_axis',(0.,0.,1.));
#20642=DIRECTION('ref_axis',(-1.,0.,0.));
#20643=DIRECTION('center_axis',(0.,0.,-1.));
#20644=DIRECTION('ref_axis',(-1.,0.,0.));
#20645=DIRECTION('center_axis',(0.,0.,-1.));
#20646=DIRECTION('ref_axis',(-1.,0.,0.));
#20647=DIRECTION('center_axis',(0.,0.,-1.));
#20648=DIRECTION('ref_axis',(-1.,0.,0.));
#20649=DIRECTION('center_axis',(0.,0.,-1.));
#20650=DIRECTION('ref_axis',(-1.,0.,0.));
#20651=DIRECTION('center_axis',(0.,0.,-1.));
#20652=DIRECTION('ref_axis',(-1.,0.,0.));
#20653=DIRECTION('center_axis',(0.,0.,-1.));
#20654=DIRECTION('ref_axis',(0.999962538604135,0.00865571420359059,0.));
#20655=DIRECTION('center_axis',(0.,0.,-1.));
#20656=DIRECTION('ref_axis',(-1.,0.,0.));
#20657=DIRECTION('center_axis',(0.,0.,-1.));
#20658=DIRECTION('ref_axis',(-1.,0.,0.));
#20659=DIRECTION('',(1.,0.,0.));
#20660=DIRECTION('',(1.,0.,0.));
#20661=DIRECTION('center_axis',(0.,0.,1.));
#20662=DIRECTION('ref_axis',(1.,0.,0.));
#20663=DIRECTION('center_axis',(0.,0.,1.));
#20664=DIRECTION('ref_axis',(1.,0.,0.));
#20665=DIRECTION('',(0.,0.,-1.));
#20666=DIRECTION('center_axis',(0.,0.,-1.));
#20667=DIRECTION('ref_axis',(1.,-5.55111512312578E-15,0.));
#20668=DIRECTION('',(0.,0.,1.));
#20669=DIRECTION('center_axis',(0.,0.,1.));
#20670=DIRECTION('ref_axis',(1.,0.,0.));
#20671=DIRECTION('center_axis',(0.,0.,1.));
#20672=DIRECTION('ref_axis',(1.,0.,0.));
#20673=DIRECTION('',(0.,0.,-1.));
#20674=DIRECTION('center_axis',(0.,0.,-1.));
#20675=DIRECTION('ref_axis',(1.,-4.16333634234433E-15,0.));
#20676=DIRECTION('',(0.,0.,1.));
#20677=DIRECTION('',(-1.,0.,0.));
#20678=DIRECTION('',(-1.,0.,0.));
#20679=DIRECTION('center_axis',(0.,0.,1.));
#20680=DIRECTION('ref_axis',(1.,0.,0.));
#20681=DIRECTION('center_axis',(0.,0.,1.));
#20682=DIRECTION('ref_axis',(-1.,0.,0.));
#20683=DIRECTION('',(0.,0.,1.));
#20684=DIRECTION('center_axis',(0.,0.,1.));
#20685=DIRECTION('ref_axis',(-1.,0.,0.));
#20686=DIRECTION('',(0.,0.,1.));
#20687=DIRECTION('center_axis',(0.,0.,1.));
#20688=DIRECTION('ref_axis',(-0.0126564647418527,-0.999919903742414,0.));
#20689=DIRECTION('center_axis',(0.,0.,-1.));
#20690=DIRECTION('ref_axis',(1.,0.,0.));
#20691=DIRECTION('',(0.,0.,1.));
#20692=DIRECTION('center_axis',(0.,0.,1.));
#20693=DIRECTION('ref_axis',(1.,0.,0.));
#20694=DIRECTION('',(0.,0.,-1.));
#20695=DIRECTION('center_axis',(0.,0.,1.));
#20696=DIRECTION('ref_axis',(1.,0.,0.));
#20697=DIRECTION('center_axis',(0.,0.,1.));
#20698=DIRECTION('ref_axis',(1.,0.,0.));
#20699=DIRECTION('',(0.,0.,1.));
#20700=DIRECTION('center_axis',(0.,0.,1.));
#20701=DIRECTION('ref_axis',(1.,0.,0.));
#20702=DIRECTION('',(0.,0.,1.));
#20703=DIRECTION('center_axis',(0.,0.,-1.));
#20704=DIRECTION('ref_axis',(-1.,0.,0.));
#20705=DIRECTION('center_axis',(0.,0.,1.));
#20706=DIRECTION('ref_axis',(1.,0.,0.));
#20707=DIRECTION('',(0.,0.,1.));
#20708=DIRECTION('',(0.,0.,1.));
#20709=DIRECTION('center_axis',(0.,0.,1.));
#20710=DIRECTION('ref_axis',(1.,0.,0.));
#20711=DIRECTION('center_axis',(0.,0.,-1.));
#20712=DIRECTION('ref_axis',(-1.,0.,0.));
#20713=DIRECTION('center_axis',(0.,0.,1.));
#20714=DIRECTION('ref_axis',(1.,0.,0.));
#20715=DIRECTION('',(0.,0.,-1.));
#20716=DIRECTION('',(0.,0.,-1.));
#20717=DIRECTION('center_axis',(0.,0.,1.));
#20718=DIRECTION('ref_axis',(1.,0.,0.));
#20719=DIRECTION('center_axis',(0.,0.,1.));
#20720=DIRECTION('ref_axis',(1.,0.,0.));
#20721=DIRECTION('center_axis',(0.,0.,1.));
#20722=DIRECTION('ref_axis',(1.,0.,0.));
#20723=DIRECTION('',(0.,0.,1.));
#20724=DIRECTION('',(0.,0.,-1.));
#20725=DIRECTION('center_axis',(0.,0.,1.));
#20726=DIRECTION('ref_axis',(1.,0.,0.));
#20727=DIRECTION('center_axis',(0.,0.,1.));
#20728=DIRECTION('ref_axis',(1.,0.,0.));
#20729=DIRECTION('center_axis',(0.,0.,1.));
#20730=DIRECTION('ref_axis',(1.,0.,0.));
#20731=DIRECTION('',(0.,0.,1.));
#20732=DIRECTION('center_axis',(0.,0.,1.));
#20733=DIRECTION('ref_axis',(1.,0.,0.));
#20734=DIRECTION('center_axis',(0.,0.,1.));
#20735=DIRECTION('ref_axis',(1.,0.,0.));
#20736=DIRECTION('',(0.,0.,1.));
#20737=DIRECTION('center_axis',(0.,0.,1.));
#20738=DIRECTION('ref_axis',(1.,0.,0.));
#20739=DIRECTION('center_axis',(0.,0.,1.));
#20740=DIRECTION('ref_axis',(1.,0.,0.));
#20741=DIRECTION('center_axis',(0.,0.,-1.));
#20742=DIRECTION('ref_axis',(1.,2.77555756156289E-15,0.));
#20743=DIRECTION('center_axis',(0.,0.,-1.));
#20744=DIRECTION('ref_axis',(1.,1.81922337360341E-15,0.));
#20745=DIRECTION('center_axis',(0.,0.,1.));
#20746=DIRECTION('ref_axis',(1.,0.,0.));
#20747=DIRECTION('center_axis',(0.,0.,1.));
#20748=DIRECTION('ref_axis',(1.,0.,0.));
#20749=DIRECTION('center_axis',(0.,0.,1.));
#20750=DIRECTION('ref_axis',(1.,0.,0.));
#20751=DIRECTION('center_axis',(0.,0.,-1.));
#20752=DIRECTION('ref_axis',(1.,0.,0.));
#20753=DIRECTION('center_axis',(0.,0.,1.));
#20754=DIRECTION('ref_axis',(1.,0.,0.));
#20755=DIRECTION('center_axis',(0.,0.,1.));
#20756=DIRECTION('ref_axis',(1.,0.,0.));
#20757=DIRECTION('center_axis',(0.,0.,-1.));
#20758=DIRECTION('ref_axis',(1.,-1.38777878078144E-15,0.));
#20759=DIRECTION('',(-0.766044443118986,0.64278760968653,0.));
#20760=DIRECTION('',(0.64278760968653,0.766044443118986,0.));
#20761=DIRECTION('center_axis',(0.,0.,1.));
#20762=DIRECTION('ref_axis',(1.,0.,0.));
#20763=DIRECTION('',(0.984807753012206,0.17364817766694,0.));
#20764=DIRECTION('',(-0.17364817766694,0.984807753012206,0.));
#20765=DIRECTION('',(0.984807753012206,0.17364817766694,0.));
#20766=DIRECTION('',(0.866025403784443,-0.499999999999992,0.));
#20767=DIRECTION('',(0.499999999999992,0.866025403784443,0.));
#20768=DIRECTION('',(0.866025403784443,-0.499999999999992,0.));
#20769=DIRECTION('center_axis',(0.,0.,1.));
#20770=DIRECTION('ref_axis',(1.,0.,0.));
#20771=DIRECTION('',(0.342020143325676,-0.939692620785906,0.));
#20772=DIRECTION('',(0.939692620785906,0.342020143325676,0.));
#20773=DIRECTION('',(0.342020143325676,-0.939692620785906,0.));
#20774=DIRECTION('center_axis',(0.,0.,1.));
#20775=DIRECTION('ref_axis',(1.,0.,0.));
#20776=DIRECTION('',(-0.342020143325663,-0.93969262078591,0.));
#20777=DIRECTION('',(0.93969262078591,-0.342020143325663,0.));
#20778=DIRECTION('',(-0.342020143325663,-0.93969262078591,0.));
#20779=DIRECTION('center_axis',(0.,0.,1.));
#20780=DIRECTION('ref_axis',(1.,0.,0.));
#20781=DIRECTION('',(-0.866025403784436,-0.500000000000004,0.));
#20782=DIRECTION('',(0.500000000000004,-0.866025403784436,0.));
#20783=DIRECTION('',(-0.866025403784436,-0.500000000000004,0.));
#20784=DIRECTION('',(0.500000000000004,-0.866025403784436,0.));
#20785=DIRECTION('center_axis',(0.,0.,1.));
#20786=DIRECTION('ref_axis',(1.,0.,0.));
#20787=DIRECTION('',(-0.173648177666927,-0.984807753012209,0.));
#20788=DIRECTION('',(-0.984807753012209,0.173648177666927,0.));
#20789=DIRECTION('',(-0.173648177666927,-0.984807753012209,0.));
#20790=DIRECTION('',(-0.984807753012209,0.173648177666927,0.));
#20791=DIRECTION('',(-0.173648177666927,-0.984807753012209,0.));
#20792=DIRECTION('center_axis',(0.,0.,1.));
#20793=DIRECTION('ref_axis',(1.,0.,0.));
#20794=DIRECTION('',(-0.64278760968654,0.766044443118977,0.));
#20795=DIRECTION('',(-0.766044443118977,-0.64278760968654,0.));
#20796=DIRECTION('',(-0.64278760968654,0.766044443118977,0.));
#20797=DIRECTION('center_axis',(0.,0.,1.));
#20798=DIRECTION('ref_axis',(1.,0.,0.));
#20799=DIRECTION('',(0.,1.,0.));
#20800=DIRECTION('',(-1.,0.,0.));
#20801=DIRECTION('',(0.,1.,0.));
#20802=DIRECTION('center_axis',(0.,0.,1.));
#20803=DIRECTION('ref_axis',(1.,0.,0.));
#20804=DIRECTION('',(0.64278760968653,0.766044443118986,0.));
#20805=DIRECTION('center_axis',(0.,0.,1.));
#20806=DIRECTION('ref_axis',(1.,0.,0.));
#20807=DIRECTION('',(0.,0.,1.));
#20808=DIRECTION('center_axis',(0.,0.,1.));
#20809=DIRECTION('ref_axis',(1.,0.,0.));
#20810=DIRECTION('',(0.,0.,1.));
#20811=DIRECTION('center_axis',(0.,0.,1.));
#20812=DIRECTION('ref_axis',(1.,0.,0.));
#20813=DIRECTION('',(0.,0.,1.));
#20814=DIRECTION('center_axis',(0.,0.,1.));
#20815=DIRECTION('ref_axis',(1.,0.,0.));
#20816=DIRECTION('',(0.,0.,1.));
#20817=DIRECTION('center_axis',(0.,0.,1.));
#20818=DIRECTION('ref_axis',(1.,0.,0.));
#20819=DIRECTION('',(0.,0.,1.));
#20820=DIRECTION('center_axis',(0.,0.,1.));
#20821=DIRECTION('ref_axis',(1.,0.,0.));
#20822=DIRECTION('',(0.,0.,1.));
#20823=DIRECTION('center_axis',(0.,0.,1.));
#20824=DIRECTION('ref_axis',(1.,0.,0.));
#20825=DIRECTION('',(0.,0.,1.));
#20826=DIRECTION('center_axis',(0.,0.,1.));
#20827=DIRECTION('ref_axis',(1.,0.,0.));
#20828=DIRECTION('',(0.,0.,1.));
#20829=DIRECTION('center_axis',(0.,0.,1.));
#20830=DIRECTION('ref_axis',(-0.988219026491317,-0.153046253402539,0.));
#20831=DIRECTION('',(0.,0.,1.));
#20832=DIRECTION('center_axis',(0.,0.,1.));
#20833=DIRECTION('ref_axis',(1.,0.,0.));
#20834=DIRECTION('',(0.,0.,-1.));
#20835=DIRECTION('center_axis',(0.,0.,1.));
#20836=DIRECTION('ref_axis',(1.,0.,0.));
#20837=DIRECTION('',(0.,0.,1.));
#20838=DIRECTION('',(0.,0.,1.));
#20839=DIRECTION('center_axis',(0.,0.,1.));
#20840=DIRECTION('ref_axis',(1.,0.,0.));
#20841=DIRECTION('center_axis',(0.,0.,1.));
#20842=DIRECTION('ref_axis',(1.,0.,0.));
#20843=DIRECTION('',(0.,0.,1.));
#20844=DIRECTION('center_axis',(0.,0.,1.));
#20845=DIRECTION('ref_axis',(1.,0.,0.));
#20846=DIRECTION('',(0.,0.,1.));
#20847=DIRECTION('center_axis',(0.,0.,1.));
#20848=DIRECTION('ref_axis',(1.,0.,0.));
#20849=DIRECTION('',(0.,0.,1.));
#20850=DIRECTION('center_axis',(0.,0.,1.));
#20851=DIRECTION('ref_axis',(1.,0.,0.));
#20852=DIRECTION('',(0.,0.,1.));
#20853=DIRECTION('center_axis',(0.,0.,1.));
#20854=DIRECTION('ref_axis',(1.,0.,0.));
#20855=DIRECTION('center_axis',(0.,0.,1.));
#20856=DIRECTION('ref_axis',(1.,0.,0.));
#20857=DIRECTION('center_axis',(0.,0.,-1.));
#20858=DIRECTION('ref_axis',(-1.,0.,0.));
#20859=DIRECTION('',(0.,0.,-1.));
#20860=DIRECTION('center_axis',(0.,0.,-1.));
#20861=DIRECTION('ref_axis',(1.,1.81922337360341E-15,0.));
#20862=DIRECTION('',(0.,0.,-1.));
#20863=DIRECTION('center_axis',(0.,0.,-1.));
#20864=DIRECTION('ref_axis',(-1.,0.,0.));
#20865=DIRECTION('center_axis',(0.,0.,1.));
#20866=DIRECTION('ref_axis',(1.,0.,0.));
#20867=DIRECTION('',(0.,0.,-1.));
#20868=DIRECTION('center_axis',(0.,0.,-1.));
#20869=DIRECTION('ref_axis',(-1.,0.,0.));
#20870=DIRECTION('center_axis',(0.,0.,1.));
#20871=DIRECTION('ref_axis',(1.,0.,0.));
#20872=DIRECTION('center_axis',(0.,0.,-1.));
#20873=DIRECTION('ref_axis',(-1.,0.,0.));
#20874=DIRECTION('center_axis',(0.,0.,-1.));
#20875=DIRECTION('ref_axis',(1.,0.,0.));
#20876=DIRECTION('',(0.,0.,-1.));
#20877=DIRECTION('center_axis',(0.,0.,-1.));
#20878=DIRECTION('ref_axis',(-1.,0.,0.));
#20879=DIRECTION('center_axis',(0.,0.,1.));
#20880=DIRECTION('ref_axis',(1.,0.,0.));
#20881=DIRECTION('',(0.,0.,-1.));
#20882=DIRECTION('center_axis',(0.,0.,-1.));
#20883=DIRECTION('ref_axis',(-1.,0.,0.));
#20884=DIRECTION('center_axis',(0.,0.,1.));
#20885=DIRECTION('ref_axis',(1.,0.,0.));
#20886=DIRECTION('',(0.,0.,1.));
#20887=DIRECTION('center_axis',(0.,0.,1.));
#20888=DIRECTION('ref_axis',(1.,0.,0.));
#20889=DIRECTION('center_axis',(0.,0.,1.));
#20890=DIRECTION('ref_axis',(1.,0.,0.));
#20891=DIRECTION('center_axis',(0.,0.,1.));
#20892=DIRECTION('ref_axis',(1.,0.,0.));
#20893=DIRECTION('center_axis',(0.,0.,1.));
#20894=DIRECTION('ref_axis',(1.,0.,0.));
#20895=DIRECTION('',(0.,1.,0.));
#20896=DIRECTION('',(-1.,0.,0.));
#20897=DIRECTION('',(0.,-1.,0.));
#20898=DIRECTION('center_axis',(0.,0.,1.));
#20899=DIRECTION('ref_axis',(1.,0.,0.));
#20900=DIRECTION('',(-0.64278760968653,-0.766044443118986,0.));
#20901=DIRECTION('',(-0.766044443118986,0.64278760968653,0.));
#20902=DIRECTION('',(-0.64278760968653,-0.766044443118986,0.));
#20903=DIRECTION('',(0.,-1.,0.));
#20904=DIRECTION('',(-1.,0.,0.));
#20905=DIRECTION('',(0.,-1.,0.));
#20906=DIRECTION('',(0.64278760968654,-0.766044443118977,0.));
#20907=DIRECTION('',(-0.766044443118977,-0.64278760968654,0.));
#20908=DIRECTION('',(0.64278760968654,-0.766044443118977,0.));
#20909=DIRECTION('',(-0.173648177666927,-0.984807753012209,0.));
#20910=DIRECTION('',(0.984807753012209,-0.173648177666927,0.));
#20911=DIRECTION('',(-0.173648177666927,-0.984807753012209,0.));
#20912=DIRECTION('',(0.984807753012209,-0.173648177666927,0.));
#20913=DIRECTION('',(-0.173648177666927,-0.984807753012209,0.));
#20914=DIRECTION('',(0.500000000000004,-0.866025403784436,0.));
#20915=DIRECTION('',(0.866025403784436,0.500000000000004,0.));
#20916=DIRECTION('',(0.500000000000004,-0.866025403784436,0.));
#20917=DIRECTION('',(0.866025403784436,0.500000000000004,0.));
#20918=DIRECTION('',(0.342020143325663,0.93969262078591,0.));
#20919=DIRECTION('',(0.93969262078591,-0.342020143325663,0.));
#20920=DIRECTION('',(0.342020143325663,0.93969262078591,0.));
#20921=DIRECTION('',(-0.342020143325676,0.939692620785906,0.));
#20922=DIRECTION('',(0.939692620785906,0.342020143325676,0.));
#20923=DIRECTION('',(-0.342020143325676,0.939692620785906,0.));
#20924=DIRECTION('',(-0.866025403784443,0.499999999999992,0.));
#20925=DIRECTION('',(0.499999999999992,0.866025403784443,0.));
#20926=DIRECTION('',(-0.866025403784443,0.499999999999992,0.));
#20927=DIRECTION('',(-0.984807753012206,-0.17364817766694,0.));
#20928=DIRECTION('',(-0.17364817766694,0.984807753012206,0.));
#20929=DIRECTION('',(-0.984807753012206,-0.17364817766694,0.));
#20930=DIRECTION('',(0.,1.,0.));
#20931=DIRECTION('',(0.,-1.,0.));
#20932=DIRECTION('',(-1.,0.,0.));
#20933=DIRECTION('center_axis',(0.,0.,1.));
#20934=DIRECTION('ref_axis',(-1.,1.45473230946492E-15,0.));
#20935=DIRECTION('center_axis',(0.,-0.152153200171805,-0.98835692119673));
#20936=DIRECTION('ref_axis',(0.,0.98835692119673,-0.152153200171805));
#20937=DIRECTION('',(0.,-0.98835692119673,0.152153200171805));
#20938=DIRECTION('',(0.,-0.98835692119673,0.152153200171805));
#20939=DIRECTION('center_axis',(-1.,0.,0.));
#20940=DIRECTION('ref_axis',(0.,0.,1.));
#20941=DIRECTION('center_axis',(-1.,0.,0.));
#20942=DIRECTION('ref_axis',(0.,0.,1.));
#20943=DIRECTION('center_axis',(0.0978021918445919,-0.11655611349438,-0.98835692119673));
#20944=DIRECTION('ref_axis',(1.08893713285454E-18,0.993118054469193,-0.117117589999644));
#20945=DIRECTION('',(0.635303582893194,-0.757125327300936,0.152153200171805));
#20946=DIRECTION('',(0.635303582893194,-0.757125327300936,0.152153200171805));
#20947=DIRECTION('center_axis',(-0.766044443118977,-0.64278760968654,0.));
#20948=DIRECTION('ref_axis',(0.,0.,1.));
#20949=DIRECTION('center_axis',(-0.766044443118977,-0.64278760968654,0.));
#20950=DIRECTION('ref_axis',(0.,0.,1.));
#20951=DIRECTION('center_axis',(-0.984807753012209,0.173648177666927,0.));
#20952=DIRECTION('ref_axis',(-0.173648177666927,-0.984807753012209,0.));
#20953=DIRECTION('',(0.,0.,-1.));
#20954=DIRECTION('center_axis',(-0.984807753012209,0.173648177666927,0.));
#20955=DIRECTION('ref_axis',(-0.173648177666927,-0.984807753012209,0.));
#20956=DIRECTION('',(0.,0.,-1.));
#20957=DIRECTION('center_axis',(0.149841651174812,-0.0264211259360251,-0.98835692119673));
#20958=DIRECTION('ref_axis',(-0.988702075986957,-2.27568915914982E-19,-0.149893978995429));
#20959=DIRECTION('',(0.973341558737816,-0.171626378250307,0.152153200171805));
#20960=DIRECTION('',(0.973341558737816,-0.171626378250307,0.152153200171805));
#20961=DIRECTION('center_axis',(-0.173648177666927,-0.984807753012209,0.));
#20962=DIRECTION('ref_axis',(0.,0.,1.));
#20963=DIRECTION('center_axis',(-0.173648177666927,-0.984807753012209,0.));
#20964=DIRECTION('ref_axis',(0.,0.,1.));
#20965=DIRECTION('center_axis',(-0.866025403784436,-0.500000000000004,0.));
#20966=DIRECTION('ref_axis',(0.500000000000004,-0.866025403784436,0.));
#20967=DIRECTION('',(0.,0.,-1.));
#20968=DIRECTION('center_axis',(0.131768536615881,0.0760766000859029,-0.98835692119673));
#20969=DIRECTION('ref_axis',(-0.991229527971275,-4.70862379419472E-20,-0.132151514852626));
#20970=DIRECTION('',(0.85594220176254,0.494178460598369,0.152153200171805));
#20971=DIRECTION('',(0.85594220176254,0.494178460598369,0.152153200171805));
#20972=DIRECTION('center_axis',(0.500000000000004,-0.866025403784436,0.));
#20973=DIRECTION('ref_axis',(0.,0.,1.));
#20974=DIRECTION('center_axis',(0.500000000000004,-0.866025403784436,0.));
#20975=DIRECTION('ref_axis',(0.,0.,1.));
#20976=DIRECTION('center_axis',(0.0520394593302189,0.142977239430406,-0.98835692119673));
#20977=DIRECTION('ref_axis',(5.2259940538791E-19,0.98969793283463,0.143171232246077));
#20978=DIRECTION('',(0.338037975844617,0.928751705551249,0.152153200171805));
#20979=DIRECTION('',(0.338037975844617,0.928751705551249,0.152153200171805));
#20980=DIRECTION('center_axis',(0.939692620785911,-0.342020143325663,0.));
#20981=DIRECTION('ref_axis',(0.,0.,1.));
#20982=DIRECTION('center_axis',(0.939692620785911,-0.342020143325663,0.));
#20983=DIRECTION('ref_axis',(0.,0.,1.));
#20984=DIRECTION('center_axis',(-0.0520394593302208,0.142977239430406,-0.98835692119673));
#20985=DIRECTION('ref_axis',(-3.0713028184418E-19,0.98969793283463,0.143171232246077));
#20986=DIRECTION('',(-0.338037975844629,0.928751705551244,0.152153200171805));
#20987=DIRECTION('',(-0.338037975844629,0.928751705551244,0.152153200171805));
#20988=DIRECTION('center_axis',(0.939692620785906,0.342020143325676,0.));
#20989=DIRECTION('ref_axis',(0.,0.,1.));
#20990=DIRECTION('center_axis',(0.939692620785906,0.342020143325676,0.));
#20991=DIRECTION('ref_axis',(0.,0.,1.));
#20992=DIRECTION('center_axis',(-0.131768536615882,0.076076600085901,-0.98835692119673));
#20993=DIRECTION('ref_axis',(-0.991229527971275,2.06899881612888E-19,0.132151514852627));
#20994=DIRECTION('',(-0.855942201762547,0.494178460598357,0.152153200171805));
#20995=DIRECTION('',(-0.855942201762547,0.494178460598357,0.152153200171805));
#20996=DIRECTION('center_axis',(0.499999999999992,0.866025403784443,0.));
#20997=DIRECTION('ref_axis',(0.,0.,1.));
#20998=DIRECTION('center_axis',(0.499999999999992,0.866025403784443,0.));
#20999=DIRECTION('ref_axis',(0.,0.,1.));
#21000=DIRECTION('center_axis',(-0.149841651174811,-0.0264211259360271,
-0.98835692119673));
#21001=DIRECTION('ref_axis',(-0.988702075986957,-4.57290035202453E-19,0.149893978995429));
#21002=DIRECTION('',(-0.973341558737814,-0.17162637825032,0.152153200171805));
#21003=DIRECTION('',(-0.973341558737814,-0.17162637825032,0.152153200171805));
#21004=DIRECTION('center_axis',(-0.17364817766694,0.984807753012206,0.));
#21005=DIRECTION('ref_axis',(0.,0.,1.));
#21006=DIRECTION('center_axis',(-0.17364817766694,0.984807753012206,0.));
#21007=DIRECTION('ref_axis',(0.,0.,1.));
#21008=DIRECTION('center_axis',(-0.0978021918445904,-0.116556113494382,
-0.98835692119673));
#21009=DIRECTION('ref_axis',(-4.42616424608758E-19,0.993118054469193,-0.117117589999646));
#21010=DIRECTION('',(-0.635303582893184,-0.757125327300944,0.152153200171805));
#21011=DIRECTION('',(-0.635303582893184,-0.757125327300944,0.152153200171805));
#21012=DIRECTION('center_axis',(-0.766044443118986,0.64278760968653,0.));
#21013=DIRECTION('ref_axis',(0.,0.,1.));
#21014=DIRECTION('center_axis',(-0.766044443118986,0.64278760968653,0.));
#21015=DIRECTION('ref_axis',(0.,0.,1.));
#21016=DIRECTION('center_axis',(0.,0.,1.));
#21017=DIRECTION('ref_axis',(-0.957942704987207,0.286959533665974,0.));
#21018=DIRECTION('center_axis',(0.,0.,1.));
#21019=DIRECTION('ref_axis',(-0.957942704987206,-0.286959533665975,0.));
#21020=DIRECTION('center_axis',(1.,0.,0.));
#21021=DIRECTION('ref_axis',(0.,0.,-1.));
#21022=DIRECTION('',(0.,0.,1.));
#21023=DIRECTION('center_axis',(-1.,0.,0.));
#21024=DIRECTION('ref_axis',(0.,0.,1.));
#21025=DIRECTION('',(0.,0.,1.));
#21026=DIRECTION('center_axis',(0.,1.,0.));
#21027=DIRECTION('ref_axis',(0.,0.,1.));
#25628=CARTESIAN_POINT('',(0.,0.,0.));
#25629=CARTESIAN_POINT('Origin',(6.93889390390723E-15,1.21430643318376E-14,
-7.));
#25630=CARTESIAN_POINT('',(-184.50486486776,-91.6185289127127,-7.));
#25631=CARTESIAN_POINT('',(-184.50486486776,91.6185289127127,-7.));
#25632=CARTESIAN_POINT('Origin',(6.93889390390723E-15,1.21430643318376E-14,
-7.));
#25633=CARTESIAN_POINT('',(-184.50486486776,91.6185289127127,-10.));
#25634=CARTESIAN_POINT('',(-184.50486486776,91.6185289127127,-7.));
#25635=CARTESIAN_POINT('',(-184.50486486776,-91.6185289127127,-10.));
#25636=CARTESIAN_POINT('Origin',(6.93889390390723E-15,1.21430643318376E-14,
-10.));
#25637=CARTESIAN_POINT('',(-184.50486486776,-91.6185289127127,-7.));
#25638=CARTESIAN_POINT('Origin',(-71.5953323638214,6.93889390390723E-15,
-7.));
#25639=CARTESIAN_POINT('Origin',(-71.5953323638214,6.93889390390723E-15,
-7.));
#25640=CARTESIAN_POINT('Origin',(-71.5953323638214,6.93889390390723E-15,
-10.));
#25641=CARTESIAN_POINT('Origin',(-210.,0.,0.));
#25642=CARTESIAN_POINT('',(-210.,-6.12323399573677E-16,5.));
#25643=CARTESIAN_POINT('Origin',(-210.,0.,0.));
#25644=CARTESIAN_POINT('',(-204.,-1.32734112397626E-14,5.));
#25645=CARTESIAN_POINT('',(-210.,-6.12323399573677E-16,5.));
#25646=CARTESIAN_POINT('',(-203.969359287593,-3.53561414983974,3.53545365999116));
#25647=CARTESIAN_POINT('Ctrl Pts',(-203.969360444161,-3.53553390593274,
3.53553390593274));
#25648=CARTESIAN_POINT('Ctrl Pts',(-203.977055116563,-3.09161865850825,
3.97944915335723));
#25649=CARTESIAN_POINT('Ctrl Pts',(-203.985248421744,-2.52939665845125,
4.36424514979789));
#25650=CARTESIAN_POINT('Ctrl Pts',(-203.996803640531,-1.29750744995471,
4.8745212692142));
#25651=CARTESIAN_POINT('Ctrl Pts',(-204.,-0.627838117491496,5.));
#25652=CARTESIAN_POINT('Ctrl Pts',(-204.,-6.93889390390723E-16,5.));
#25653=CARTESIAN_POINT('',(-203.938716194739,-4.99999958112187,0.00204287664667749));
#25654=CARTESIAN_POINT('Ctrl Pts',(-203.938716295296,-4.99999958266548,
0.00204287664629751));
#25655=CARTESIAN_POINT('Ctrl Pts',(-203.938722578506,-4.99974330468984,
0.629290622414902));
#25656=CARTESIAN_POINT('Ctrl Pts',(-203.941919986053,-4.87424456118115,
1.29817546531228));
#25657=CARTESIAN_POINT('Ctrl Pts',(-203.953470693038,-4.36427603534107,
2.52932209840595));
#25658=CARTESIAN_POINT('Ctrl Pts',(-203.961663784593,-3.97954354876496,
3.09148377916774));
#25659=CARTESIAN_POINT('Ctrl Pts',(-203.969357649916,-3.53569510571298,
3.53537269880239));
#25660=CARTESIAN_POINT('',(-203.969331848638,-3.53718156034075,-3.53388548308072));
#25661=CARTESIAN_POINT('Ctrl Pts',(-203.96933187763,-3.5371815607091,-3.53388548294644));
#25662=CARTESIAN_POINT('Ctrl Pts',(-203.961645461725,-3.98041386013988,
-3.09023977789374));
#25663=CARTESIAN_POINT('Ctrl Pts',(-203.953464241805,-4.36456085996178,
-2.52863448563173));
#25664=CARTESIAN_POINT('Ctrl Pts',(-203.941913718727,-4.87452126623505,
-1.29750745448768));
#25665=CARTESIAN_POINT('Ctrl Pts',(-203.938716285064,-5.,-0.627838125135884));
#25666=CARTESIAN_POINT('Ctrl Pts',(-203.938716285064,-5.,0.));
#25667=CARTESIAN_POINT('Ctrl Pts',(-203.938716285064,-5.,0.000680909716903597));
#25668=CARTESIAN_POINT('Ctrl Pts',(-203.938716288475,-4.99999986090858,
0.00136186863985322));
#25669=CARTESIAN_POINT('Ctrl Pts',(-203.938716295296,-4.99999958266548,
0.00204287664629765));
#25670=CARTESIAN_POINT('',(-203.99999999855,-0.000260375111436809,-4.99999993829161));
#25671=CARTESIAN_POINT('Ctrl Pts',(-203.999999999834,-0.000260375114298633,
-4.99999999322048));
#25672=CARTESIAN_POINT('Ctrl Pts',(-203.99999919859,-0.628023263685998,
-4.99996730245366));
#25673=CARTESIAN_POINT('Ctrl Pts',(-203.996802841847,-1.29759259672811,
-4.87448599951234));
#25674=CARTESIAN_POINT('Ctrl Pts',(-203.985248421744,-2.52939665845125,
-4.36424514979789));
#25675=CARTESIAN_POINT('Ctrl Pts',(-203.977055116563,-3.09161865850825,
-3.97944915335723));
#25676=CARTESIAN_POINT('Ctrl Pts',(-203.969350922768,-3.53608320695274,
-3.53498460491273));
#25677=CARTESIAN_POINT('Ctrl Pts',(-203.969341400589,-3.53663242527553,
-3.53443513056216));
#25678=CARTESIAN_POINT('Ctrl Pts',(-203.96933187763,-3.5371815607091,-3.53388548294644));
#25679=CARTESIAN_POINT('',(-203.969412573458,3.53252077317422,-3.53854447085706));
#25680=CARTESIAN_POINT('Ctrl Pts',(-203.969412650463,3.53252077489201,-3.53854447124186));
#25681=CARTESIAN_POINT('Ctrl Pts',(-203.977092222053,3.0890986957704,-3.98121170893611));
#25682=CARTESIAN_POINT('Ctrl Pts',(-203.985261486298,2.52800386071199,-4.36482207783705));
#25683=CARTESIAN_POINT('Ctrl Pts',(-203.996803640531,1.29750744995471,-4.8745212692142));
#25684=CARTESIAN_POINT('Ctrl Pts',(-204.,0.627838117491497,-5.));
#25685=CARTESIAN_POINT('Ctrl Pts',(-204.,1.11022302462516E-15,-5.));
#25686=CARTESIAN_POINT('',(-203.938716348762,4.99999732701828,-0.00517006110607621));
#25687=CARTESIAN_POINT('Ctrl Pts',(-203.938716350598,4.9999973270461,-0.0051700611060565));
#25688=CARTESIAN_POINT('Ctrl Pts',(-203.938732229062,4.99934967998715,-0.631513444132154));
#25689=CARTESIAN_POINT('Ctrl Pts',(-203.94192957817,4.87382106523366,-1.29919785313323));
#25690=CARTESIAN_POINT('Ctrl Pts',(-203.953471392542,4.36424515196542,-2.52939665587767));
#25691=CARTESIAN_POINT('Ctrl Pts',(-203.961665771665,3.97944915876222,-3.09161865310325));
#25692=CARTESIAN_POINT('Ctrl Pts',(-203.969377843651,3.53453010762235,-3.53653770424313));
#25693=CARTESIAN_POINT('Ctrl Pts',(-203.969395245763,3.53352573047557,-3.53754122640331));
#25694=CARTESIAN_POINT('Ctrl Pts',(-203.969412650463,3.53252077489201,-3.53854447124186));
#25695=CARTESIAN_POINT('',(-203.969318710503,3.53793517768081,3.53313100014201));
#25696=CARTESIAN_POINT('Ctrl Pts',(-203.969318807181,3.53793517953451,3.53313100031857));
#25697=CARTESIAN_POINT('Ctrl Pts',(-203.961636172418,3.98085504657878,3.08960887244123));
#25698=CARTESIAN_POINT('Ctrl Pts',(-203.953460970419,4.3647052930154,2.52828580084305));
#25699=CARTESIAN_POINT('Ctrl Pts',(-203.941913718727,4.87452126623505,1.29750745448768));
#25700=CARTESIAN_POINT('Ctrl Pts',(-203.938716285064,5.,0.627838125135884));
#25701=CARTESIAN_POINT('Ctrl Pts',(-203.938716285064,5.,-0.00172303923949561));
#25702=CARTESIAN_POINT('Ctrl Pts',(-203.938716306901,4.99999910934032,-0.00344639360360825));
#25703=CARTESIAN_POINT('Ctrl Pts',(-203.938716350598,4.9999973270461,-0.0051700611060567));
#25704=CARTESIAN_POINT('Ctrl Pts',(-204.,-4.16333634234434E-16,5.));
#25705=CARTESIAN_POINT('Ctrl Pts',(-204.,0.627838117491495,5.));
#25706=CARTESIAN_POINT('Ctrl Pts',(-203.996803640531,1.29750744995471,4.8745212692142));
#25707=CARTESIAN_POINT('Ctrl Pts',(-203.985248421744,2.52939665845125,4.36424514979789));
#25708=CARTESIAN_POINT('Ctrl Pts',(-203.977055116563,3.09161865850825,3.97944915335723));
#25709=CARTESIAN_POINT('Ctrl Pts',(-203.969346566832,3.53633450633251,3.53473330553297));
#25710=CARTESIAN_POINT('Ctrl Pts',(-203.969332687833,3.53713493106456,3.53393233692737));
#25711=CARTESIAN_POINT('Ctrl Pts',(-203.969318807181,3.53793517953451,3.53313100031857));
#25712=CARTESIAN_POINT('Origin',(-71.5953323638214,6.93889390390723E-15,
10.));
#25713=CARTESIAN_POINT('',(-174.6884520924,105.356275112407,10.));
#25714=CARTESIAN_POINT('',(-174.6884520924,-105.356275112407,10.));
#25715=CARTESIAN_POINT('Origin',(-71.5953323638214,6.93889390390723E-15,
10.));
#25716=CARTESIAN_POINT('',(-174.6884520924,105.356275112407,-10.));
#25717=CARTESIAN_POINT('',(-174.6884520924,105.356275112407,10.));
#25718=CARTESIAN_POINT('',(-174.6884520924,-105.356275112407,-10.));
#25719=CARTESIAN_POINT('Origin',(-71.5953323638214,6.93889390390723E-15,
-10.));
#25720=CARTESIAN_POINT('',(-174.6884520924,-105.356275112407,10.));
#25721=CARTESIAN_POINT('Origin',(-35.7976661819107,9.54097911787244E-15,
-10.));
#25722=CARTESIAN_POINT('Origin',(6.93889390390723E-15,1.21430643318376E-14,
-10.));
#25723=CARTESIAN_POINT('Origin',(-35.7976661819107,9.54097911787244E-15,
10.));
#25724=CARTESIAN_POINT('Origin',(6.93889390390723E-15,1.21430643318376E-14,
10.));
#25725=CARTESIAN_POINT('',(-184.50486486776,91.6185289127127,10.));
#25726=CARTESIAN_POINT('',(-184.50486486776,-91.6185289127127,10.));
#25727=CARTESIAN_POINT('Origin',(-71.5953323638214,6.93889390390723E-15,
10.));
#25728=CARTESIAN_POINT('Origin',(6.93889390390723E-15,1.21430643318376E-14,
10.));
#25729=CARTESIAN_POINT('Origin',(-210.,0.,0.));
#25730=CARTESIAN_POINT('Origin',(-71.5953323638214,6.93889390390723E-15,
7.));
#25731=CARTESIAN_POINT('',(-184.50486486776,-91.6185289127127,7.));
#25732=CARTESIAN_POINT('',(-184.50486486776,-91.6185289127127,7.));
#25733=CARTESIAN_POINT('',(-184.50486486776,91.6185289127127,7.));
#25734=CARTESIAN_POINT('Origin',(-71.5953323638214,6.93889390390723E-15,
7.));
#25735=CARTESIAN_POINT('',(-184.50486486776,91.6185289127127,7.));
#25736=CARTESIAN_POINT('Origin',(6.93889390390723E-15,1.21430643318376E-14,
7.));
#25737=CARTESIAN_POINT('Origin',(6.93889390390723E-15,1.21430643318376E-14,
7.));
#25738=CARTESIAN_POINT('Origin',(-35.7976661819107,9.54097911787244E-15,
7.));
#25739=CARTESIAN_POINT('Origin',(-35.7976661819107,9.54097911787244E-15,
-7.));
#25740=CARTESIAN_POINT('Origin',(6.93889390390723E-15,1.21430643318376E-14,
12.5));
#25741=CARTESIAN_POINT('Ctrl Pts',(-203.969357610281,-3.53569510523211,
3.53537269900855));
#25742=CARTESIAN_POINT('Ctrl Pts',(-203.969356693716,-3.53574798064454,
3.53531981895734));
#25743=CARTESIAN_POINT('Ctrl Pts',(-203.969355777146,-3.53580085486419,
3.53526693763481));
#25744=CARTESIAN_POINT('Ctrl Pts',(-203.969354860571,-3.53585372789099,
3.53521405504099));
#25745=CARTESIAN_POINT('Ctrl Pts',(-203.969353523271,-3.5359308706626,3.53513689831092));
#25746=CARTESIAN_POINT('Ctrl Pts',(-203.969352185979,-3.53600801081182,
3.5350597388574));
#25747=CARTESIAN_POINT('Ctrl Pts',(-203.969350848697,-3.53608514833853,
3.53498257668063));
#25748=CARTESIAN_POINT('Ctrl Pts',(-203.968102971582,-3.60806555270628,
3.46297917027145));
#25749=CARTESIAN_POINT('Ctrl Pts',(-203.966863395218,-3.67743065556072,
3.38894263048284));
#25750=CARTESIAN_POINT('Ctrl Pts',(-203.965637313051,-3.74428389561946,
3.31295292278655));
#25751=CARTESIAN_POINT('Ctrl Pts',(-203.964393266827,-3.81211664212436,
3.23584984484127));
#25752=CARTESIAN_POINT('Ctrl Pts',(-203.963163096211,-3.877363644099,3.15673552555768));
#25753=CARTESIAN_POINT('Ctrl Pts',(-203.961952291397,-3.94009625713642,
3.07565384174656));
#25754=CARTESIAN_POINT('Ctrl Pts',(-203.960730121248,-4.00341771586461,
2.99381107693147));
#25755=CARTESIAN_POINT('Ctrl Pts',(-203.959527664023,-4.06417763323105,
2.90996337813423));
#25756=CARTESIAN_POINT('Ctrl Pts',(-203.958350897716,-4.122408262698,2.82412250980142));
#25757=CARTESIAN_POINT('Ctrl Pts',(-203.957172007328,-4.18074399933042,
2.73812669740508));
#25758=CARTESIAN_POINT('Ctrl Pts',(-203.956018882071,-4.23654156600736,
2.65013001319041));
#25759=CARTESIAN_POINT('Ctrl Pts',(-203.954898139835,-4.28978839858892,
2.56011827232567));
#25760=CARTESIAN_POINT('Ctrl Pts',(-203.953783867703,-4.34272783439241,
2.47062617399722));
#25761=CARTESIAN_POINT('Ctrl Pts',(-203.952701587561,-4.39314613126717,
2.37914170259479));
#25762=CARTESIAN_POINT('Ctrl Pts',(-203.951658676823,-4.44098296523244,
2.28563285085449));
#25763=CARTESIAN_POINT('Ctrl Pts',(-203.950633072017,-4.48802600064509,
2.19367567352523));
#25764=CARTESIAN_POINT('Ctrl Pts',(-203.949645524783,-4.53257269388454,
2.09976023710277));
#25765=CARTESIAN_POINT('Ctrl Pts',(-203.948704148847,-4.57451641576525,
2.00384615015072));
#25766=CARTESIAN_POINT('Ctrl Pts',(-203.948404891615,-4.58785004969342,
1.97335569134953));
#25767=CARTESIAN_POINT('Ctrl Pts',(-203.948110309694,-4.60092024898877,
1.94266321081319));
#25768=CARTESIAN_POINT('Ctrl Pts',(-203.947820691679,-4.61372247670505,
1.91176732253888));
#25769=CARTESIAN_POINT('Ctrl Pts',(-203.946912093852,-4.65388598749793,
1.81483986821907));
#25770=CARTESIAN_POINT('Ctrl Pts',(-203.946063611632,-4.6907675717227,1.7174757848906));
#25771=CARTESIAN_POINT('Ctrl Pts',(-203.945278888644,-4.7244863460725,1.61972835506864));
#25772=CARTESIAN_POINT('Ctrl Pts',(-203.944484940015,-4.75860153715152,
1.5208317519103));
#25773=CARTESIAN_POINT('Ctrl Pts',(-203.943756240949,-4.78947932184167,
1.42154221971967));
#25774=CARTESIAN_POINT('Ctrl Pts',(-203.94309699481,-4.81719984076717,1.32188335555093));
#25775=CARTESIAN_POINT('Ctrl Pts',(-203.942432162295,-4.84515526023121,
1.22137999345174));
#25776=CARTESIAN_POINT('Ctrl Pts',(-203.941837946665,-4.8698998937537,1.12050048682021));
#25777=CARTESIAN_POINT('Ctrl Pts',(-203.941319364095,-4.89146906173073,
1.01924502824124));
#25778=CARTESIAN_POINT('Ctrl Pts',(-203.941232999844,-4.89506117054544,
1.00238204003108));
#25779=CARTESIAN_POINT('Ctrl Pts',(-203.941148735228,-4.89856509815127,
0.985508581542827));
#25780=CARTESIAN_POINT('Ctrl Pts',(-203.941066595844,-4.90198087606653,
0.968624605516958));
#25781=CARTESIAN_POINT('Ctrl Pts',(-203.94063972183,-4.91973249253479,0.880879478548298));
#25782=CARTESIAN_POINT('Ctrl Pts',(-203.94027118057,-4.9350824150589,0.79297491825541));
#25783=CARTESIAN_POINT('Ctrl Pts',(-203.939960217077,-4.94804802325662,
0.704798382938753));
#25784=CARTESIAN_POINT('Ctrl Pts',(-203.939651507015,-4.9609196747494,0.617260828577294));
#25785=CARTESIAN_POINT('Ctrl Pts',(-203.939399529957,-4.97144155245078,
0.52945478342709));
#25786=CARTESIAN_POINT('Ctrl Pts',(-203.939204733522,-4.97958027609786,
0.44126268565492));
#25787=CARTESIAN_POINT('Ctrl Pts',(-203.9390135821,-4.9875667087051,0.354720830212983));
#25788=CARTESIAN_POINT('Ctrl Pts',(-203.938877480764,-4.99325838390049,
0.267806829941029));
#25789=CARTESIAN_POINT('Ctrl Pts',(-203.938798171246,-4.99657408274633,
0.180408643921277));
#25790=CARTESIAN_POINT('Ctrl Pts',(-203.938744615543,-4.99881308995086,
0.12139086900888));
#25791=CARTESIAN_POINT('Ctrl Pts',(-203.938716983673,-4.99996764782323,
0.062152291453425));
#25792=CARTESIAN_POINT('Ctrl Pts',(-203.938716201879,-4.99999929267631,
0.00265955567477993));
#25793=CARTESIAN_POINT('Ctrl Pts',(-203.938716200513,-4.99999934795696,
0.00255562733875602));
#25794=CARTESIAN_POINT('Ctrl Pts',(-203.938716199228,-4.99999939986611,
0.00245169825933746));
#25795=CARTESIAN_POINT('Ctrl Pts',(-203.938716198025,-4.99999944840367,
0.00234776843634019));
#25796=CARTESIAN_POINT('Ctrl Pts',(-203.938716196848,-4.99999949586766,
0.00224613737482393));
#25797=CARTESIAN_POINT('Ctrl Pts',(-203.938716195753,-4.99999954010701,
0.00214450677827265));
#25798=CARTESIAN_POINT('Ctrl Pts',(-203.938716194739,-4.99999958112187,
0.00204287664667743));
#25799=CARTESIAN_POINT('Origin',(6.93889390390723E-15,1.21430643318376E-14,
12.5));
#25800=CARTESIAN_POINT('Ctrl Pts',(-204.,-1.32734112397625E-14,5.));
#25801=CARTESIAN_POINT('Ctrl Pts',(-204.,-0.105934998674852,5.));
#25802=CARTESIAN_POINT('Ctrl Pts',(-203.999905939126,-0.211337971606702,
4.99651966715266));
#25803=CARTESIAN_POINT('Ctrl Pts',(-203.999725729962,-0.316230501501799,
4.98968355835091));
#25804=CARTESIAN_POINT('Ctrl Pts',(-203.999538700243,-0.425093003726101,
4.98258871651251));
#25805=CARTESIAN_POINT('Ctrl Pts',(-203.999258867793,-0.533406187565095,
4.9718793685295));
#25806=CARTESIAN_POINT('Ctrl Pts',(-203.998893507736,-0.64119150817493,
4.95763708121322));
#25807=CARTESIAN_POINT('Ctrl Pts',(-203.998532826796,-0.74759643673455,
4.94357719294793));
#25808=CARTESIAN_POINT('Ctrl Pts',(-203.998088773486,-0.853487399797586,
4.92607394237269));
#25809=CARTESIAN_POINT('Ctrl Pts',(-203.997567101389,-0.958875298258525,
4.90515317922688));
#25810=CARTESIAN_POINT('Ctrl Pts',(-203.997045990193,-1.0641498837675,4.8842549100625));
#25811=CARTESIAN_POINT('Ctrl Pts',(-203.996447409029,-1.16892297110147,
4.85994627755904));
#25812=CARTESIAN_POINT('Ctrl Pts',(-203.995776131441,-1.27318855674928,
4.8322039916926));
#25813=CARTESIAN_POINT('Ctrl Pts',(-203.995109685905,-1.37670360839317,
4.80466140286675));
#25814=CARTESIAN_POINT('Ctrl Pts',(-203.994371568543,-1.47971891143702,
4.77373420137415));
#25815=CARTESIAN_POINT('Ctrl Pts',(-203.993565773266,-1.58220484941587,
4.73935434229579));
#25816=CARTESIAN_POINT('Ctrl Pts',(-203.992732918314,-1.68813240120964,
4.70381996192122));
#25817=CARTESIAN_POINT('Ctrl Pts',(-203.991827746257,-1.79349523021465,
4.66459724220142));
#25818=CARTESIAN_POINT('Ctrl Pts',(-203.990854206795,-1.89822529428719,
4.62156297086283));
#25819=CARTESIAN_POINT('Ctrl Pts',(-203.990755308256,-1.90886446274436,
4.61719126665108));
#25820=CARTESIAN_POINT('Ctrl Pts',(-203.990655669341,-1.91950065693411,
4.61277864479938));
#25821=CARTESIAN_POINT('Ctrl Pts',(-203.990555535075,-1.93010846927917,
4.60833566613732));
#25822=CARTESIAN_POINT('Ctrl Pts',(-203.989623947544,-2.02879702187669,
4.56700092914183));
#25823=CARTESIAN_POINT('Ctrl Pts',(-203.988645783478,-2.12544454260582,
4.52287513049451));
#25824=CARTESIAN_POINT('Ctrl Pts',(-203.987628217859,-2.22009981897521,
4.47607498314025));
#25825=CARTESIAN_POINT('Ctrl Pts',(-203.986576674134,-2.31791578307618,
4.4277121056641));
#25826=CARTESIAN_POINT('Ctrl Pts',(-203.985483038528,-2.41360478322964,
4.3764932632756));
#25827=CARTESIAN_POINT('Ctrl Pts',(-203.984353960946,-2.50720785336269,
4.32249107453453));
#25828=CARTESIAN_POINT('Ctrl Pts',(-203.983224883364,-2.60081092349573,
4.26848888579346));
#25829=CARTESIAN_POINT('Ctrl Pts',(-203.982060342399,-2.69232855862323,
4.21170304388256));
#25830=CARTESIAN_POINT('Ctrl Pts',(-203.980866027979,-2.78178136197962,
4.15215395164811));
#25831=CARTESIAN_POINT('Ctrl Pts',(-203.977955208569,-2.99979845363451,
4.00701909379552));
#25832=CARTESIAN_POINT('Ctrl Pts',(-203.974852066525,-3.20665944575788,
3.84469935011728));
#25833=CARTESIAN_POINT('Ctrl Pts',(-203.97166383987,-3.39947681026973,3.66637359289185));
#25834=CARTESIAN_POINT('Ctrl Pts',(-203.970899480465,-3.44570368867466,
3.62362099580809));
#25835=CARTESIAN_POINT('Ctrl Pts',(-203.970130239275,-3.49112317575354,
3.5799485388053));
#25836=CARTESIAN_POINT('Ctrl Pts',(-203.969357610281,-3.53569510523211,
3.53537269900855));
#25837=CARTESIAN_POINT('Origin',(6.93889390390723E-15,1.21430643318376E-14,
12.5));
#25838=CARTESIAN_POINT('Ctrl Pts',(-203.969318710503,3.53793517768081,3.53313100014201));
#25839=CARTESIAN_POINT('Ctrl Pts',(-203.969319343331,3.53789869384933,3.53316753322899));
#25840=CARTESIAN_POINT('Ctrl Pts',(-203.969319976156,3.53786220936332,3.53320406579359));
#25841=CARTESIAN_POINT('Ctrl Pts',(-203.969320608979,3.53782572422278,3.53324059783579));
#25842=CARTESIAN_POINT('Ctrl Pts',(-203.970611807987,3.46338221651318,3.60777980269651));
#25843=CARTESIAN_POINT('Ctrl Pts',(-203.971888843469,3.38684047652641,3.67952299153842));
#25844=CARTESIAN_POINT('Ctrl Pts',(-203.973147340404,3.30828782941231,3.7485675397376));
#25845=CARTESIAN_POINT('Ctrl Pts',(-203.974474867646,3.22542646040027,3.8213992773911));
#25846=CARTESIAN_POINT('Ctrl Pts',(-203.975781787315,3.14032736598223,3.89122878189774));
#25847=CARTESIAN_POINT('Ctrl Pts',(-203.977062936614,3.05304750252111,3.95812848589098));
#25848=CARTESIAN_POINT('Ctrl Pts',(-203.978344085913,2.96576763905998,4.02502818988422));
#25849=CARTESIAN_POINT('Ctrl Pts',(-203.979599486566,2.87630643596515,4.08899834926344));
#25850=CARTESIAN_POINT('Ctrl Pts',(-203.980823625848,2.78468276933246,4.15006483737447));
#25851=CARTESIAN_POINT('Ctrl Pts',(-203.981870899358,2.70629704939164,4.20230833308643));
#25852=CARTESIAN_POINT('Ctrl Pts',(-203.982894364117,2.62639950599981,4.2523802263174));
#25853=CARTESIAN_POINT('Ctrl Pts',(-203.983891257211,2.54490943418125,4.30032213736983));
#25854=CARTESIAN_POINT('Ctrl Pts',(-203.984884418463,2.46372441826546,4.3480845791614));
#25855=CARTESIAN_POINT('Ctrl Pts',(-203.985851223315,2.38095835588121,4.39373317038848));
#25856=CARTESIAN_POINT('Ctrl Pts',(-203.986788196368,2.29650898991706,4.43726262079967));
#25857=CARTESIAN_POINT('Ctrl Pts',(-203.987715596661,2.21292241663634,4.48034734446959));
#25858=CARTESIAN_POINT('Ctrl Pts',(-203.98861378765,2.12768634428916,4.52135620175186));
#25859=CARTESIAN_POINT('Ctrl Pts',(-203.989478428242,2.04068579461556,4.56023551915283));
#25860=CARTESIAN_POINT('Ctrl Pts',(-203.989733389213,2.01503149991839,4.57170006127321));
#25861=CARTESIAN_POINT('Ctrl Pts',(-203.989985425568,1.98922369851592,4.58297910210696));
#25862=CARTESIAN_POINT('Ctrl Pts',(-203.990234406414,1.96325925710145,4.59407040651396));
#25863=CARTESIAN_POINT('Ctrl Pts',(-203.990344101315,1.95181995613283,4.59895696529723));
#25864=CARTESIAN_POINT('Ctrl Pts',(-203.990453202995,1.9403502493567,4.60380707787955));
#25865=CARTESIAN_POINT('Ctrl Pts',(-203.990561699649,1.92884986487884,4.6086205279904));
#25866=CARTESIAN_POINT('Ctrl Pts',(-203.99064911369,1.91958418678222,4.61249864870428));
#25867=CARTESIAN_POINT('Ctrl Pts',(-203.990736158426,1.91029601075009,4.61635400051938));
#25868=CARTESIAN_POINT('Ctrl Pts',(-203.99082262093,1.90100758274172,4.62017734818583));
#25869=CARTESIAN_POINT('Ctrl Pts',(-203.9917505584,1.80132182385841,4.66121048245372));
#25870=CARTESIAN_POINT('Ctrl Pts',(-203.992616459951,1.70108357376192,4.69878322677367));
#25871=CARTESIAN_POINT('Ctrl Pts',(-203.993417023432,1.60035035707351,4.73300773477725));
#25872=CARTESIAN_POINT('Ctrl Pts',(-203.994226939003,1.49844038654684,4.76763204954248));
#25873=CARTESIAN_POINT('Ctrl Pts',(-203.994969999376,1.39602334141336,4.79882966441702));
#25874=CARTESIAN_POINT('Ctrl Pts',(-203.99564238175,1.29312684702631,4.8266737670285));
#25875=CARTESIAN_POINT('Ctrl Pts',(-203.996333096745,1.18742486192691,4.8552770439125));
#25876=CARTESIAN_POINT('Ctrl Pts',(-203.996949249375,1.08121648770143,4.88034184081964));
#25877=CARTESIAN_POINT('Ctrl Pts',(-203.997485958936,0.974505079806989,
4.90189757804557));
#25878=CARTESIAN_POINT('Ctrl Pts',(-203.998010132875,0.870286070072518,
4.92294985007637));
#25879=CARTESIAN_POINT('Ctrl Pts',(-203.998458545774,0.765586677755228,
4.94065505980157));
#25880=CARTESIAN_POINT('Ctrl Pts',(-203.998825695445,0.660392869034546,
4.95499142144511));
#25881=CARTESIAN_POINT('Ctrl Pts',(-203.999206015696,0.551425494589673,
4.96984206433358));
#25882=CARTESIAN_POINT('Ctrl Pts',(-203.999499166199,0.441927125126886,
4.98107840366953));
#25883=CARTESIAN_POINT('Ctrl Pts',(-203.999697656623,0.331871235928197,
4.98861781341002));
#25884=CARTESIAN_POINT('Ctrl Pts',(-203.999884886851,0.228058725888239,
4.99572951869974));
#25885=CARTESIAN_POINT('Ctrl Pts',(-203.999987896713,0.123749676165767,
4.99955156729294));
#25886=CARTESIAN_POINT('Ctrl Pts',(-203.999998997644,0.0189194210330657,
4.99996287881259));
#25887=CARTESIAN_POINT('Ctrl Pts',(-203.999999665264,0.0126148337550222,
4.99998761546301));
#25888=CARTESIAN_POINT('Ctrl Pts',(-204.,0.00630836177732318,5.));
#25889=CARTESIAN_POINT('Ctrl Pts',(-204.,1.11022302462516E-14,5.));
#25890=CARTESIAN_POINT('Origin',(6.93889390390723E-15,1.21430643318376E-14,
12.5));
#25891=CARTESIAN_POINT('Ctrl Pts',(-203.938716348762,4.99999732701828,-0.00517006110607632));
#25892=CARTESIAN_POINT('Ctrl Pts',(-203.93871634805,4.99999735605216,-0.00514200020558854));
#25893=CARTESIAN_POINT('Ctrl Pts',(-203.938716347344,4.99999738484058,-0.00511393926482346));
#25894=CARTESIAN_POINT('Ctrl Pts',(-203.938716346644,4.99999741338354,-0.00508587828380103));
#25895=CARTESIAN_POINT('Ctrl Pts',(-203.938716346556,4.9999974169859,-0.00508233675359046));
#25896=CARTESIAN_POINT('Ctrl Pts',(-203.938716346468,4.99999742058435,-0.00507879522309794));
#25897=CARTESIAN_POINT('Ctrl Pts',(-203.93871634638,4.9999974241789,-0.0050752536923105));
#25898=CARTESIAN_POINT('Ctrl Pts',(-203.938713709765,5.0001049778899,0.100892144113212));
#25899=CARTESIAN_POINT('Ctrl Pts',(-203.938799494166,4.99671862708652,0.206347959533171));
#25900=CARTESIAN_POINT('Ctrl Pts',(-203.938967699789,4.98996531629572,0.311310410519268));
#25901=CARTESIAN_POINT('Ctrl Pts',(-203.939138036895,4.98312642831378,0.417602933822402));
#25902=CARTESIAN_POINT('Ctrl Pts',(-203.939392912403,4.97283458317559,0.52338996686812));
#25903=CARTESIAN_POINT('Ctrl Pts',(-203.939727564256,4.95916798069977,0.628688768458106));
#25904=CARTESIAN_POINT('Ctrl Pts',(-203.940073274326,4.94504977977268,0.737467057784966));
#25905=CARTESIAN_POINT('Ctrl Pts',(-203.940504132557,4.92733017598478,0.84572488698958));
#25906=CARTESIAN_POINT('Ctrl Pts',(-203.941016241189,4.90603868496409,0.953471599031184));
#25907=CARTESIAN_POINT('Ctrl Pts',(-203.941515990555,4.88526104432011,1.0586179441695));
#25908=CARTESIAN_POINT('Ctrl Pts',(-203.942093138348,4.86108144605084,1.16327799154476));
#25909=CARTESIAN_POINT('Ctrl Pts',(-203.942745048659,4.83347748759248,1.26744392065104));
#25910=CARTESIAN_POINT('Ctrl Pts',(-203.943421142492,4.80484952178682,1.37547403021185));
#25911=CARTESIAN_POINT('Ctrl Pts',(-203.944177664023,4.77253855205537,1.48297343929525));
#25912=CARTESIAN_POINT('Ctrl Pts',(-203.945012471915,4.73646667417703,1.58990607313729));
#25913=CARTESIAN_POINT('Ctrl Pts',(-203.945800498774,4.70241619508238,1.69084640747349));
#25914=CARTESIAN_POINT('Ctrl Pts',(-203.94665830582,4.66501394975628,1.79128196025224));
#25915=CARTESIAN_POINT('Ctrl Pts',(-203.947584499091,4.62415254700364,1.89115185460711));
#25916=CARTESIAN_POINT('Ctrl Pts',(-203.94763948234,4.62172681931875,1.89708060769205));
#25917=CARTESIAN_POINT('Ctrl Pts',(-203.947694706664,4.61928888940156,1.90300735722081));
#25918=CARTESIAN_POINT('Ctrl Pts',(-203.947750171796,4.61683873043373,1.90893208653466));
#25919=CARTESIAN_POINT('Ctrl Pts',(-203.948683491776,4.57560954282768,2.00862838363326));
#25920=CARTESIAN_POINT('Ctrl Pts',(-203.949669808962,4.53153795147535,2.1062639160333));
#25921=CARTESIAN_POINT('Ctrl Pts',(-203.950699952284,4.48474857734145,2.20187922861786));
#25922=CARTESIAN_POINT('Ctrl Pts',(-203.951742583665,4.43739199240551,2.29865365134534));
#25923=CARTESIAN_POINT('Ctrl Pts',(-203.952830128236,4.38725112293232,2.39335905712821));
#25924=CARTESIAN_POINT('Ctrl Pts',(-203.953954290108,4.33440264927066,2.4860269299219));
#25925=CARTESIAN_POINT('Ctrl Pts',(-203.955118538022,4.27966967288282,2.58199920957561));
#25926=CARTESIAN_POINT('Ctrl Pts',(-203.956322077217,4.2220325491105,2.6757866843588));
#25927=CARTESIAN_POINT('Ctrl Pts',(-203.957556728966,4.16152180946428,2.76740444721753));
#25928=CARTESIAN_POINT('Ctrl Pts',(-203.958753673601,4.1028591094598,2.85622414053291));
#25929=CARTESIAN_POINT('Ctrl Pts',(-203.959979882541,4.0414951366038,2.94300498366657));
#25930=CARTESIAN_POINT('Ctrl Pts',(-203.961228553297,3.97741192006286,3.02773540654414));
#25931=CARTESIAN_POINT('Ctrl Pts',(-203.962468242802,3.91378963162541,3.11185639320373));
#25932=CARTESIAN_POINT('Ctrl Pts',(-203.963730090487,3.84748681331452,3.19395678144878));
#25933=CARTESIAN_POINT('Ctrl Pts',(-203.965007789759,3.77844536602085,3.27399396499808));
#25934=CARTESIAN_POINT('Ctrl Pts',(-203.966265184082,3.71050111200704,3.35275921316117));
#25935=CARTESIAN_POINT('Ctrl Pts',(-203.967537947166,3.63990430694283,3.42952667847006));
#25936=CARTESIAN_POINT('Ctrl Pts',(-203.968820147925,3.56656423888803,3.50421953305103));
#25937=CARTESIAN_POINT('Ctrl Pts',(-203.968983759641,3.55720588040194,3.51375051015614));
#25938=CARTESIAN_POINT('Ctrl Pts',(-203.969147524933,3.54780281043576,3.52324765428997));
#25939=CARTESIAN_POINT('Ctrl Pts',(-203.969311431355,3.53835480166774,3.53271075769229));
#25940=CARTESIAN_POINT('Ctrl Pts',(-203.969313857769,3.53821493662746,3.5328508461883));
#25941=CARTESIAN_POINT('Ctrl Pts',(-203.969316284151,3.53807506196518,3.53299092700489));
#25942=CARTESIAN_POINT('Ctrl Pts',(-203.969318710503,3.53793517768081,3.53313100014201));
#25943=CARTESIAN_POINT('Origin',(6.93889390390723E-15,1.21430643318376E-14,
12.5));
#25944=CARTESIAN_POINT('Ctrl Pts',(-203.969412573458,3.53252077317421,-3.53854447085706));
#25945=CARTESIAN_POINT('Ctrl Pts',(-203.969411275839,3.53259569826288,-3.53846967256236));
#25946=CARTESIAN_POINT('Ctrl Pts',(-203.96940997822,3.53267062140505,-3.53839487125771));
#25947=CARTESIAN_POINT('Ctrl Pts',(-203.969408680599,3.53274554260078,-3.53832006694293));
#25948=CARTESIAN_POINT('Ctrl Pts',(-203.968134468,3.60631520091507,-3.4648651811077));
#25949=CARTESIAN_POINT('Ctrl Pts',(-203.966868845506,3.67715439213078,-3.38936634640809));
#25950=CARTESIAN_POINT('Ctrl Pts',(-203.965617535976,3.74536448123347,-3.31190366563091));
#25951=CARTESIAN_POINT('Ctrl Pts',(-203.964349534112,3.81448448556256,-3.23340764105307));
#25952=CARTESIAN_POINT('Ctrl Pts',(-203.963096212182,3.88090503780374,-3.15289462678018));
#25953=CARTESIAN_POINT('Ctrl Pts',(-203.96186354839,3.94469528542177,-3.07040827976421));
#25954=CARTESIAN_POINT('Ctrl Pts',(-203.960558807129,4.01221553602298,-2.98309871396592));
#25955=CARTESIAN_POINT('Ctrl Pts',(-203.959277185763,4.07678958330119,-2.8935780934403));
#25956=CARTESIAN_POINT('Ctrl Pts',(-203.958026129452,4.13845115188194,-2.80185832588414));
#25957=CARTESIAN_POINT('Ctrl Pts',(-203.956833143225,4.19725058518819,-2.71439590026936));
#25958=CARTESIAN_POINT('Ctrl Pts',(-203.955667935116,4.25340153535253,-2.62493301863032));
#25959=CARTESIAN_POINT('Ctrl Pts',(-203.954537560927,4.30688757918469,-2.53345274735351));
#25960=CARTESIAN_POINT('Ctrl Pts',(-203.953413583761,4.36007093438034,-2.44249018194157));
#25961=CARTESIAN_POINT('Ctrl Pts',(-203.952324028895,4.41061969182416,-2.34953252211284));
#25962=CARTESIAN_POINT('Ctrl Pts',(-203.951276693114,4.4584700718099,-2.25454397745184));
#25963=CARTESIAN_POINT('Ctrl Pts',(-203.950245015845,4.50560505011277,-2.16097558796462));
#25964=CARTESIAN_POINT('Ctrl Pts',(-203.949254288028,4.55012190726754,-2.06543612011637));
#25965=CARTESIAN_POINT('Ctrl Pts',(-203.948313055999,4.59191045159328,-1.9678797168031));
#25966=CARTESIAN_POINT('Ctrl Pts',(-203.948147566562,4.59925780322778,-1.95072714039958));
#25967=CARTESIAN_POINT('Ctrl Pts',(-203.947983610346,4.60652068476313,-1.93351219424609));
#25968=CARTESIAN_POINT('Ctrl Pts',(-203.94782123798,4.613698330089,-1.91623460785442));
#25969=CARTESIAN_POINT('Ctrl Pts',(-203.946900124353,4.65441601552921,-1.81822149966598));
#25970=CARTESIAN_POINT('Ctrl Pts',(-203.946045172056,4.69176958275255,-1.71969832859259));
#25971=CARTESIAN_POINT('Ctrl Pts',(-203.945257471353,4.72587584163911,-1.62071281896581));
#25972=CARTESIAN_POINT('Ctrl Pts',(-203.944460536852,4.76038191014495,-1.52056695460618));
#25973=CARTESIAN_POINT('Ctrl Pts',(-203.943732421809,4.7915643076881,-1.41994737344693));
#25974=CARTESIAN_POINT('Ctrl Pts',(-203.943074663623,4.81950096756316,-1.31887158134935));
#25975=CARTESIAN_POINT('Ctrl Pts',(-203.942413007084,4.84760320038007,-1.21719674067824));
#25976=CARTESIAN_POINT('Ctrl Pts',(-203.941822525777,4.87242131004307,-1.11505977428861));
#25977=CARTESIAN_POINT('Ctrl Pts',(-203.941305468174,4.8939882340887,-1.01245374825097));
#25978=CARTESIAN_POINT('Ctrl Pts',(-203.940789741936,4.91549962575811,-0.910111921059155));
#25979=CARTESIAN_POINT('Ctrl Pts',(-203.940347044837,4.93377671234906,-0.807302952881646));
#25980=CARTESIAN_POINT('Ctrl Pts',(-203.939980546822,4.94880355906628,-0.704002840896675));
#25981=CARTESIAN_POINT('Ctrl Pts',(-203.939616664476,4.96372316028913,-0.601439974175979));
#25982=CARTESIAN_POINT('Ctrl Pts',(-203.93932788155,4.97543889374863,-0.498392480078721));
#25983=CARTESIAN_POINT('Ctrl Pts',(-203.939118470203,4.98388497402619,-0.394827141948199));
#25984=CARTESIAN_POINT('Ctrl Pts',(-203.938912457629,4.99219397340393,-0.292942681724858));
#25985=CARTESIAN_POINT('Ctrl Pts',(-203.938783247807,4.99733867728785,-0.190556617638261));
#25986=CARTESIAN_POINT('Ctrl Pts',(-203.938736256528,4.99920612957307,-0.0876345386283712));
#25987=CARTESIAN_POINT('Ctrl Pts',(-203.938723723722,4.99970418832119,-0.0601847118080584));
#25988=CARTESIAN_POINT('Ctrl Pts',(-203.938717047394,4.9999688458647,-0.0326967616464312));
#25989=CARTESIAN_POINT('Ctrl Pts',(-203.938716348762,4.99999732701828,-0.00517006110607632));
#25990=CARTESIAN_POINT('Origin',(6.93889390390723E-15,1.21430643318376E-14,
12.5));
#25991=CARTESIAN_POINT('Ctrl Pts',(-203.999999998715,-4.1209657214436E-14,
-4.99999998173599));
#25992=CARTESIAN_POINT('Ctrl Pts',(-203.999999851572,0.101478108507438,
-4.99999789027357));
#25993=CARTESIAN_POINT('Ctrl Pts',(-203.999911491604,0.202547192110731,
-4.99673137395367));
#25994=CARTESIAN_POINT('Ctrl Pts',(-203.999742496303,0.303223851399144,
-4.99032853877155));
#25995=CARTESIAN_POINT('Ctrl Pts',(-203.999570703464,0.405567105534984,
-4.9838197114737));
#25996=CARTESIAN_POINT('Ctrl Pts',(-203.999315569935,0.507505311344336,
-4.97406977581446));
#25997=CARTESIAN_POINT('Ctrl Pts',(-203.998983564952,0.60905786453182,-4.96115979848574));
#25998=CARTESIAN_POINT('Ctrl Pts',(-203.998647122097,0.711967858954138,
-4.94807725498299));
#25999=CARTESIAN_POINT('Ctrl Pts',(-203.998231724043,0.814482346588999,
-4.93174952421542));
#26000=CARTESIAN_POINT('Ctrl Pts',(-203.997742803152,0.916615882329558,
-4.91220799556483));
#26001=CARTESIAN_POINT('Ctrl Pts',(-203.997253924647,1.01874056404149,-4.89266816098322));
#26002=CARTESIAN_POINT('Ctrl Pts',(-203.996691518543,1.12048489244614,-4.8699148964471));
#26003=CARTESIAN_POINT('Ctrl Pts',(-203.996059973582,1.22184988589826,-4.84392933565863));
#26004=CARTESIAN_POINT('Ctrl Pts',(-203.995432907184,1.32249605576609,-4.81812804986796));
#26005=CARTESIAN_POINT('Ctrl Pts',(-203.994737661213,1.42276877071541,-4.78913993588124));
#26006=CARTESIAN_POINT('Ctrl Pts',(-203.993977768997,1.52264788095545,-4.75690006435692));
#26007=CARTESIAN_POINT('Ctrl Pts',(-203.993228127426,1.62117966161722,-4.72509509591093));
#26008=CARTESIAN_POINT('Ctrl Pts',(-203.992415554537,1.71932887167901,-4.69012528273805));
#26009=CARTESIAN_POINT('Ctrl Pts',(-203.991542958962,1.81704812208673,-4.65188621442636));
#26010=CARTESIAN_POINT('Ctrl Pts',(-203.991352020189,1.83843075833679,-4.6435188550285));
#26011=CARTESIAN_POINT('Ctrl Pts',(-203.991158206183,1.85979268381466,-4.6349948061121));
#26012=CARTESIAN_POINT('Ctrl Pts',(-203.990961545547,1.88113318328502,-4.62631271594245));
#26013=CARTESIAN_POINT('Ctrl Pts',(-203.990885740832,1.88935908201384,-4.62296612161418));
#26014=CARTESIAN_POINT('Ctrl Pts',(-203.990809513162,1.89758179638646,-4.61959604470624));
#26015=CARTESIAN_POINT('Ctrl Pts',(-203.990732864159,1.90580128199572,-4.61620240419527));
#26016=CARTESIAN_POINT('Ctrl Pts',(-203.990664473972,1.91313513024385,-4.61317442340677));
#26017=CARTESIAN_POINT('Ctrl Pts',(-203.990595782027,1.92046277100155,-4.61012917130543));
#26018=CARTESIAN_POINT('Ctrl Pts',(-203.990526862118,1.92777665320724,-4.60706983383067));
#26019=CARTESIAN_POINT('Ctrl Pts',(-203.98961484747,2.02456099013266,-4.56658573241935));
#26020=CARTESIAN_POINT('Ctrl Pts',(-203.988659330757,2.11933307478242,-4.52347601725412));
#26021=CARTESIAN_POINT('Ctrl Pts',(-203.987667121574,2.21213936003649,-4.47785962810522));
#26022=CARTESIAN_POINT('Ctrl Pts',(-203.986663494819,2.30601358783902,-4.43171832102921));
#26023=CARTESIAN_POINT('Ctrl Pts',(-203.985622308448,2.39787702616031,-4.38301209941167));
#26024=CARTESIAN_POINT('Ctrl Pts',(-203.984549391421,2.48776893667968,-4.33181135199818));
#26025=CARTESIAN_POINT('Ctrl Pts',(-203.983467856286,2.57838289563658,-4.28019933932782));
#26026=CARTESIAN_POINT('Ctrl Pts',(-203.982354060498,2.66699405089007,-4.22605234310404));
#26027=CARTESIAN_POINT('Ctrl Pts',(-203.981213017644,2.75362587927287,-4.16939260747491));
#26028=CARTESIAN_POINT('Ctrl Pts',(-203.981096128022,2.76250053427264,-4.16358832496728));
#26029=CARTESIAN_POINT('Ctrl Pts',(-203.980978951783,2.7713543994495,-4.15775763221893));
#26030=CARTESIAN_POINT('Ctrl Pts',(-203.980861493872,2.78018748681088,-4.15190052529389));
#26031=CARTESIAN_POINT('Ctrl Pts',(-203.979859088338,2.85557053765398,-4.10191499123766));
#26032=CARTESIAN_POINT('Ctrl Pts',(-203.978837504642,2.92934542439754,-4.05007367992567));
#26033=CARTESIAN_POINT('Ctrl Pts',(-203.977798594993,3.00159775461004,-3.99631196514068));
#26034=CARTESIAN_POINT('Ctrl Pts',(-203.976767279042,3.07332197106984,-3.94294321070539));
#26035=CARTESIAN_POINT('Ctrl Pts',(-203.975718873857,3.14354620234686,-3.88768178534922));
#26036=CARTESIAN_POINT('Ctrl Pts',(-203.974654798023,3.21232371174674,-3.83042363989903));
#26037=CARTESIAN_POINT('Ctrl Pts',(-203.973610516975,3.27982176716291,-3.77423065605377));
#26038=CARTESIAN_POINT('Ctrl Pts',(-203.972551128472,3.34592674794902,-3.71611429378542));
#26039=CARTESIAN_POINT('Ctrl Pts',(-203.971477814882,3.4106543595515,-3.65594048143801));
#26040=CARTESIAN_POINT('Ctrl Pts',(-203.970797314893,3.45169282156614,-3.61778920949765));
#26041=CARTESIAN_POINT('Ctrl Pts',(-203.970111214813,3.49217690578241,-3.57881018648497));
#26042=CARTESIAN_POINT('Ctrl Pts',(-203.969419821476,3.53210224850348,-3.53896223575735));
#26043=CARTESIAN_POINT('Ctrl Pts',(-203.969417405474,3.53224176347508,-3.53882299122405));
#26044=CARTESIAN_POINT('Ctrl Pts',(-203.969414989468,3.53238127169852,-3.53868373625768));
#26045=CARTESIAN_POINT('Ctrl Pts',(-203.969412573458,3.53252077317421,-3.53854447085706));
#26046=CARTESIAN_POINT('Origin',(6.93889390390723E-15,1.21430643318376E-14,
12.5));
#26047=CARTESIAN_POINT('Ctrl Pts',(-203.969331848638,-3.53718156034075,
-3.53388548308073));
#26048=CARTESIAN_POINT('Ctrl Pts',(-203.96933263622,-3.53713614484727,-3.53393094079166));
#26049=CARTESIAN_POINT('Ctrl Pts',(-203.969333423798,-3.53709072838883,
-3.53397639765148));
#26050=CARTESIAN_POINT('Ctrl Pts',(-203.969334211371,-3.53704531096541,
-3.53402185366019));
#26051=CARTESIAN_POINT('Ctrl Pts',(-203.970636762969,-3.46193033865401,
-3.60920064143309));
#26052=CARTESIAN_POINT('Ctrl Pts',(-203.971924002428,-3.38470365609248,
-3.68152944605214));
#26053=CARTESIAN_POINT('Ctrl Pts',(-203.97319187132,-3.30544129092278,-3.75111104527892));
#26054=CARTESIAN_POINT('Ctrl Pts',(-203.974475554871,-3.22519025314963,
-3.82156056487008));
#26055=CARTESIAN_POINT('Ctrl Pts',(-203.975739398606,-3.14285202075756,
-3.88919414923696));
#26056=CARTESIAN_POINT('Ctrl Pts',(-203.976979043182,-3.05846905612516,
-3.95407910561204));
#26057=CARTESIAN_POINT('Ctrl Pts',(-203.978255220119,-2.97159932320146,
-4.02087622343817));
#26058=CARTESIAN_POINT('Ctrl Pts',(-203.979505771654,-2.8825621978443,-4.08476074195069));
#26059=CARTESIAN_POINT('Ctrl Pts',(-203.980725493441,-2.7913714701466,-4.14575947632592));
#26060=CARTESIAN_POINT('Ctrl Pts',(-203.981919492977,-2.70210382915404,
-4.20547183150373));
#26061=CARTESIAN_POINT('Ctrl Pts',(-203.983083965809,-2.61077188188111,
-4.26241888838065));
#26062=CARTESIAN_POINT('Ctrl Pts',(-203.984213332899,-2.51736531855809,
-4.31657884047884));
#26063=CARTESIAN_POINT('Ctrl Pts',(-203.985379194806,-2.42094037839488,
-4.37248893881155));
#26064=CARTESIAN_POINT('Ctrl Pts',(-203.98650767288,-2.32230412745077,-4.42542946900403));
#26065=CARTESIAN_POINT('Ctrl Pts',(-203.98759153748,-2.22142770237638,-4.47532051437978));
#26066=CARTESIAN_POINT('Ctrl Pts',(-203.988619493194,-2.12575477637829,
-4.52263803468924));
#26067=CARTESIAN_POINT('Ctrl Pts',(-203.989607328797,-2.02806626724635,
-4.5672123814815));
#26068=CARTESIAN_POINT('Ctrl Pts',(-203.990547667339,-1.92832974439805,
-4.60892427326972));
#26069=CARTESIAN_POINT('Ctrl Pts',(-203.990598810864,-1.92290523271829,
-4.61119291706969));
#26070=CARTESIAN_POINT('Ctrl Pts',(-203.990649813556,-1.91747466197154,
-4.61345308059517));
#26071=CARTESIAN_POINT('Ctrl Pts',(-203.990700674109,-1.91203802672089,
-4.61570474017852));
#26072=CARTESIAN_POINT('Ctrl Pts',(-203.991624460392,-1.8132917723089,-4.65660190171607));
#26073=CARTESIAN_POINT('Ctrl Pts',(-203.992487633228,-1.71401719948977,
-4.69408846950362));
#26074=CARTESIAN_POINT('Ctrl Pts',(-203.993287114536,-1.61426436199689,
-4.72828343912112));
#26075=CARTESIAN_POINT('Ctrl Pts',(-203.994094953937,-1.51346866902538,
-4.76283589642822));
#26076=CARTESIAN_POINT('Ctrl Pts',(-203.994837780494,-1.41218417208542,
-4.79402774654659));
#26077=CARTESIAN_POINT('Ctrl Pts',(-203.995511933048,-1.31043346085766,
-4.8219370383235));
#26078=CARTESIAN_POINT('Ctrl Pts',(-203.996191074818,-1.20792972070238,
-4.85005287906505));
#26079=CARTESIAN_POINT('Ctrl Pts',(-203.996800540141,-1.10495234407624,
-4.8748375765012));
#26080=CARTESIAN_POINT('Ctrl Pts',(-203.997335830203,-1.00150255967545,
-4.89632312555432));
#26081=CARTESIAN_POINT('Ctrl Pts',(-203.997390348359,-0.990966418640601,
-4.89851138313596));
#26082=CARTESIAN_POINT('Ctrl Pts',(-203.997444096318,-0.98042536252555,
-4.90066537665444));
#26083=CARTESIAN_POINT('Ctrl Pts',(-203.997497068777,-0.969879383161346,
-4.90278511114707));
#26084=CARTESIAN_POINT('Ctrl Pts',(-203.998675482326,-0.735275867146641,
-4.94994025414655));
#26085=CARTESIAN_POINT('Ctrl Pts',(-203.999475416986,-0.497158016437222,
-4.98036087920727));
#26086=CARTESIAN_POINT('Ctrl Pts',(-203.99981546314,-0.257667439114993,
-4.99312496300635));
#26087=CARTESIAN_POINT('Ctrl Pts',(-203.999936376277,-0.172509714040374,
-4.99766359810066));
#26088=CARTESIAN_POINT('Ctrl Pts',(-203.999999125432,-0.0871786927026717,
-4.99996942432042));
#26089=CARTESIAN_POINT('Ctrl Pts',(-203.999999989755,-0.00177162224212113,
-4.99999968613545));
#26090=CARTESIAN_POINT('Ctrl Pts',(-203.999999992743,-0.0014763523465126,
-4.9999997907568));
#26091=CARTESIAN_POINT('Ctrl Pts',(-203.999999994983,-0.00118108191426726,
-4.99999986769981));
#26092=CARTESIAN_POINT('Ctrl Pts',(-203.999999996477,-0.000885810949727572,
-4.99999991696603));
#26093=CARTESIAN_POINT('Origin',(6.93889390390723E-15,1.21430643318376E-14,
12.5));
#26094=CARTESIAN_POINT('Ctrl Pts',(-203.938716194739,-4.99999958112187,
0.00204287664667743));
#26095=CARTESIAN_POINT('Ctrl Pts',(-203.938715152034,-5.0000417830682,-0.102528719030479));
#26096=CARTESIAN_POINT('Ctrl Pts',(-203.938800539213,-4.99667457281812,
-0.206607538294783));
#26097=CARTESIAN_POINT('Ctrl Pts',(-203.938966293367,-4.99002608380757,
-0.310206534216836));
#26098=CARTESIAN_POINT('Ctrl Pts',(-203.939134229435,-4.98329007704069,
-0.415169261306567));
#26099=CARTESIAN_POINT('Ctrl Pts',(-203.939384676877,-4.9731857396949,-0.519639916075042));
#26100=CARTESIAN_POINT('Ctrl Pts',(-203.93971286547,-4.95979262703873,-0.623634161057456));
#26101=CARTESIAN_POINT('Ctrl Pts',(-203.940057644038,-4.94572249081783,
-0.732885328478902));
#26102=CARTESIAN_POINT('Ctrl Pts',(-203.940488230322,-4.92802295076255,
-0.841611316229411));
#26103=CARTESIAN_POINT('Ctrl Pts',(-203.941000611062,-4.90672556926535,
-0.949824308092555));
#26104=CARTESIAN_POINT('Ctrl Pts',(-203.941492763979,-4.88626896810742,
-1.0537652557129));
#26105=CARTESIAN_POINT('Ctrl Pts',(-203.942060406374,-4.86249247252813,
-1.15723335870826));
#26106=CARTESIAN_POINT('Ctrl Pts',(-203.94270105974,-4.83537271866045,-1.26022634082892));
#26107=CARTESIAN_POINT('Ctrl Pts',(-203.94333810678,-4.80840562560068,-1.36263956135086));
#26108=CARTESIAN_POINT('Ctrl Pts',(-203.944047362564,-4.77813263765291,
-1.46458349161457));
#26109=CARTESIAN_POINT('Ctrl Pts',(-203.944827171486,-4.74448357436985,
-1.56603569119861));
#26110=CARTESIAN_POINT('Ctrl Pts',(-203.945595488905,-4.71133037405031,
-1.66599285991305));
#26111=CARTESIAN_POINT('Ctrl Pts',(-203.946432312624,-4.67489966245849,
-1.76547313517111));
#26112=CARTESIAN_POINT('Ctrl Pts',(-203.947336562213,-4.63508122875481,
-1.86442843748819));
#26113=CARTESIAN_POINT('Ctrl Pts',(-203.947474281927,-4.62901677113549,
-1.87949960381216));
#26114=CARTESIAN_POINT('Ctrl Pts',(-203.947613566339,-4.6228736522463,-1.89455853425889));
#26115=CARTESIAN_POINT('Ctrl Pts',(-203.947754412286,-4.61665139773073,
-1.90960499330604));
#26116=CARTESIAN_POINT('Ctrl Pts',(-203.948679171294,-4.57579764205161,
-2.00839625300285));
#26117=CARTESIAN_POINT('Ctrl Pts',(-203.949656115491,-4.5321554336636,-2.10515411801173));
#26118=CARTESIAN_POINT('Ctrl Pts',(-203.950676240678,-4.48584283790299,
-2.19992344521772));
#26119=CARTESIAN_POINT('Ctrl Pts',(-203.951708300859,-4.43898840613736,
-2.29580152983209));
#26120=CARTESIAN_POINT('Ctrl Pts',(-203.952784575849,-4.38940055633292,
-2.38964476280578));
#26121=CARTESIAN_POINT('Ctrl Pts',(-203.953897000685,-4.3371485721777,-2.48149181013575));
#26122=CARTESIAN_POINT('Ctrl Pts',(-203.955064903076,-4.28229073797331,
-2.57791934635375));
#26123=CARTESIAN_POINT('Ctrl Pts',(-203.956272663953,-4.22449658832434,
-2.67214732123704));
#26124=CARTESIAN_POINT('Ctrl Pts',(-203.957512102244,-4.16378789801569,
-2.76420269877084));
#26125=CARTESIAN_POINT('Ctrl Pts',(-203.958696582427,-4.10577110031478,
-2.85217623581319));
#26126=CARTESIAN_POINT('Ctrl Pts',(-203.95991001783,-4.04509190437419,-2.93816590008804));
#26127=CARTESIAN_POINT('Ctrl Pts',(-203.961145986998,-3.98172187707493,
-3.02217234792129));
#26128=CARTESIAN_POINT('Ctrl Pts',(-203.962373099065,-3.91880596694053,
-3.10557679554172));
#26129=CARTESIAN_POINT('Ctrl Pts',(-203.963622440477,-3.85323742532754,
-3.18702678160715));
#26130=CARTESIAN_POINT('Ctrl Pts',(-203.964888151834,-3.78494613139692,
-3.26649414243936));
#26131=CARTESIAN_POINT('Ctrl Pts',(-203.966133891314,-3.71773241754321,
-3.34470757411209));
#26132=CARTESIAN_POINT('Ctrl Pts',(-203.967395504321,-3.64788095752727,
-3.42100082378285));
#26133=CARTESIAN_POINT('Ctrl Pts',(-203.968667570102,-3.57528732430931,
-3.49531319775564));
#26134=CARTESIAN_POINT('Ctrl Pts',(-203.968887824704,-3.56271794143041,
-3.50818017574942));
#26135=CARTESIAN_POINT('Ctrl Pts',(-203.96910839275,-3.5500662608768,-3.52098767609423));
#26136=CARTESIAN_POINT('Ctrl Pts',(-203.969329246069,-3.53733163160961,
-3.53373526569466));
#26137=CARTESIAN_POINT('Ctrl Pts',(-203.969330113598,-3.5372816090241,-3.53378533918933));
#26138=CARTESIAN_POINT('Ctrl Pts',(-203.969330981121,-3.53723158526782,
-3.53383541165135));
#26139=CARTESIAN_POINT('Ctrl Pts',(-203.969331848638,-3.53718156034075,
-3.53388548308073));
#26140=CARTESIAN_POINT('Origin',(-6.93889390390723E-15,1.21430643318376E-14,
7.));
#26141=CARTESIAN_POINT('',(184.50486486776,-91.6185289127127,7.));
#26142=CARTESIAN_POINT('',(184.50486486776,91.6185289127127,7.));
#26143=CARTESIAN_POINT('Origin',(-6.93889390390723E-15,1.21430643318376E-14,
7.));
#26144=CARTESIAN_POINT('',(184.50486486776,91.6185289127127,10.));
#26145=CARTESIAN_POINT('',(184.50486486776,91.6185289127127,7.));
#26146=CARTESIAN_POINT('',(184.50486486776,-91.6185289127127,10.));
#26147=CARTESIAN_POINT('Origin',(-6.93889390390723E-15,1.21430643318376E-14,
10.));
#26148=CARTESIAN_POINT('',(184.50486486776,-91.6185289127127,7.));
#26149=CARTESIAN_POINT('Origin',(71.5953323638214,6.93889390390723E-15,
7.));
#26150=CARTESIAN_POINT('Origin',(71.5953323638214,6.93889390390723E-15,
7.));
#26151=CARTESIAN_POINT('Origin',(71.5953323638214,6.93889390390723E-15,
10.));
#26152=CARTESIAN_POINT('Origin',(210.,0.,0.));
#26153=CARTESIAN_POINT('',(210.,-6.12323399573677E-16,-5.));
#26154=CARTESIAN_POINT('Origin',(210.,0.,0.));
#26155=CARTESIAN_POINT('',(204.000000000871,-0.000351443158057461,-4.9999996843097));
#26156=CARTESIAN_POINT('',(210.,-6.12323399573677E-16,-5.));
#26157=CARTESIAN_POINT('',(203.969329275182,-3.53733162599185,-3.53373527131814));
#26158=CARTESIAN_POINT('Ctrl Pts',(203.969329275182,-3.53733162599185,-3.53373527131814));
#26159=CARTESIAN_POINT('Ctrl Pts',(203.969339665773,-3.53673248458769,-3.53433502248076));
#26160=CARTESIAN_POINT('Ctrl Pts',(203.969350055435,-3.53613324448486,-3.53493456738062));
#26161=CARTESIAN_POINT('Ctrl Pts',(203.977055116563,-3.09161865850825,-3.97944915335723));
#26162=CARTESIAN_POINT('Ctrl Pts',(203.985248421744,-2.52939665845125,-4.36424514979789));
#26163=CARTESIAN_POINT('Ctrl Pts',(203.996801483377,-1.29773742182364,-4.87442600971193));
#26164=CARTESIAN_POINT('Ctrl Pts',(203.999997835124,-0.628338172338108,
-4.99991167307061));
#26165=CARTESIAN_POINT('Ctrl Pts',(203.999999998788,-0.000703254944229431,
-4.99999995054325));
#26166=CARTESIAN_POINT('',(203.938716302406,-4.99999929267631,0.00265955567476925));
#26167=CARTESIAN_POINT('Ctrl Pts',(203.938716302406,-4.99999929267631,0.00265955567477076));
#26168=CARTESIAN_POINT('Ctrl Pts',(203.938716290844,-4.99999976426973,0.00177295390105103));
#26169=CARTESIAN_POINT('Ctrl Pts',(203.938716285064,-5.,0.000886435252659898));
#26170=CARTESIAN_POINT('Ctrl Pts',(203.938716285064,-5.,-0.627838125135884));
#26171=CARTESIAN_POINT('Ctrl Pts',(203.941913718727,-4.87452126623505,-1.29750745448768));
#26172=CARTESIAN_POINT('Ctrl Pts',(203.953463590422,-4.36458961878151,-2.52856505718217));
#26173=CARTESIAN_POINT('Ctrl Pts',(203.961643611968,-3.98050171479364,-3.09011415925124));
#26174=CARTESIAN_POINT('Ctrl Pts',(203.969329275182,-3.53733162599185,-3.53373527131814));
#26175=CARTESIAN_POINT('',(203.969357682308,-3.53569323348296,3.53537456396855));
#26176=CARTESIAN_POINT('Ctrl Pts',(203.969354900228,-3.535853727891,3.53521405504098));
#26177=CARTESIAN_POINT('Ctrl Pts',(203.961661829301,-3.97963642785498,3.09135105562694));
#26178=CARTESIAN_POINT('Ctrl Pts',(203.953470004699,-4.36430642577637,2.52924873097206));
#26179=CARTESIAN_POINT('Ctrl Pts',(203.94192187778,-4.87416104063058,1.29837709745118));
#26180=CARTESIAN_POINT('Ctrl Pts',(203.938724479991,-4.99966574739792,0.629729021401888));
#26181=CARTESIAN_POINT('Ctrl Pts',(203.938716302406,-4.99999929267631,0.00265955567477064));
#26182=CARTESIAN_POINT('',(204.,1.86713497344704E-14,5.));
#26183=CARTESIAN_POINT('Ctrl Pts',(204.,2.77555756156289E-16,5.));
#26184=CARTESIAN_POINT('Ctrl Pts',(204.,-0.627838117491495,5.));
#26185=CARTESIAN_POINT('Ctrl Pts',(203.996803640531,-1.29750744995471,4.8745212692142));
#26186=CARTESIAN_POINT('Ctrl Pts',(203.985248421744,-2.52939665845125,4.36424514979789));
#26187=CARTESIAN_POINT('Ctrl Pts',(203.977055116563,-3.09161865850825,3.97944915335723));
#26188=CARTESIAN_POINT('Ctrl Pts',(203.969360444161,-3.53553390593274,3.53553390593274));
#26189=CARTESIAN_POINT('',(203.969311528224,3.5383548016686,3.53271075769143));
#26190=CARTESIAN_POINT('Ctrl Pts',(203.969311528224,3.5383548016686,3.53271075769143));
#26191=CARTESIAN_POINT('Ctrl Pts',(203.969327835823,3.53741474617601,3.53365231506597));
#26192=CARTESIAN_POINT('Ctrl Pts',(203.969344141145,3.53647444727618,3.53459336458929));
#26193=CARTESIAN_POINT('Ctrl Pts',(203.977055116563,3.09161865850825,3.97944915335723));
#26194=CARTESIAN_POINT('Ctrl Pts',(203.985248421744,2.52939665845125,4.36424514979789));
#26195=CARTESIAN_POINT('Ctrl Pts',(203.996803640531,1.29750744995471,4.8745212692142));
#26196=CARTESIAN_POINT('Ctrl Pts',(204.,0.627838117491496,5.));
#26197=CARTESIAN_POINT('Ctrl Pts',(204.,2.77555756156289E-16,5.));
#26198=CARTESIAN_POINT('',(203.938716348481,4.99999741338323,-0.00508587858850655));
#26199=CARTESIAN_POINT('Ctrl Pts',(203.938716348481,4.99999741338323,-0.00508587858850455));
#26200=CARTESIAN_POINT('Ctrl Pts',(203.938716306196,4.99999913810376,-0.00339028203939836));
#26201=CARTESIAN_POINT('Ctrl Pts',(203.938716285064,5.,-0.00169498854628657));
#26202=CARTESIAN_POINT('Ctrl Pts',(203.938716285064,5.,0.));
#26203=CARTESIAN_POINT('Ctrl Pts',(203.938716285064,5.,0.627838125135885));
#26204=CARTESIAN_POINT('Ctrl Pts',(203.941913718727,4.87452126623505,1.29750745448768));
#26205=CARTESIAN_POINT('Ctrl Pts',(203.953459148684,4.36478572336839,2.52809162894172));
#26206=CARTESIAN_POINT('Ctrl Pts',(203.961631000106,3.98110068786657,3.08925751744615));
#26207=CARTESIAN_POINT('Ctrl Pts',(203.969311528224,3.5383548016686,3.53271075769143));
#26208=CARTESIAN_POINT('',(203.96941989844,3.5321022485035,-3.53896223575733));
#26209=CARTESIAN_POINT('Ctrl Pts',(203.96941989844,3.5321022485035,-3.53896223575733));
#26210=CARTESIAN_POINT('Ctrl Pts',(203.96940007698,3.53324688460997,-3.53781981843381));
#26211=CARTESIAN_POINT('Ctrl Pts',(203.969380258871,3.53439077061651,-3.53667704124896));
#26212=CARTESIAN_POINT('Ctrl Pts',(203.961665771665,3.97944915876222,-3.09161865310326));
#26213=CARTESIAN_POINT('Ctrl Pts',(203.953471392542,4.36424515196542,-2.52939665587767));
#26214=CARTESIAN_POINT('Ctrl Pts',(203.941929319981,4.87383246434926,-1.29917033382159));
#26215=CARTESIAN_POINT('Ctrl Pts',(203.938731969008,4.9993602870002,-0.631453616573415));
#26216=CARTESIAN_POINT('Ctrl Pts',(203.938716348481,4.99999741338323,-0.00508587858850454));
#26217=CARTESIAN_POINT('Ctrl Pts',(204.,-4.16333634234434E-16,-5.));
#26218=CARTESIAN_POINT('Ctrl Pts',(204.,0.627838117491495,-5.));
#26219=CARTESIAN_POINT('Ctrl Pts',(203.996803640531,1.29750744995471,-4.8745212692142));
#26220=CARTESIAN_POINT('Ctrl Pts',(203.985263299786,2.52781052678752,-4.3649021610816));
#26221=CARTESIAN_POINT('Ctrl Pts',(203.977097370854,3.08874883332667,-3.98145624679971));
#26222=CARTESIAN_POINT('Ctrl Pts',(203.96941989844,3.5321022485035,-3.53896223575733));
#26223=CARTESIAN_POINT('Origin',(71.5953323638214,6.93889390390723E-15,
-10.));
#26224=CARTESIAN_POINT('',(174.6884520924,105.356275112407,-10.));
#26225=CARTESIAN_POINT('',(174.6884520924,-105.356275112407,-10.));
#26226=CARTESIAN_POINT('Origin',(71.5953323638214,6.93889390390723E-15,
-10.));
#26227=CARTESIAN_POINT('',(174.6884520924,105.356275112407,10.));
#26228=CARTESIAN_POINT('',(174.6884520924,105.356275112407,-10.));
#26229=CARTESIAN_POINT('',(174.6884520924,-105.356275112407,10.));
#26230=CARTESIAN_POINT('Origin',(71.5953323638214,6.93889390390723E-15,
10.));
#26231=CARTESIAN_POINT('',(174.6884520924,-105.356275112407,-10.));
#26232=CARTESIAN_POINT('Origin',(35.7976661819107,9.54097911787244E-15,
10.));
#26233=CARTESIAN_POINT('',(204.,-1.28397303707684E-14,10.));
#26234=CARTESIAN_POINT('Origin',(6.93889390390723E-15,1.21430643318376E-14,
10.));
#26235=CARTESIAN_POINT('Origin',(6.93889390390723E-15,1.21430643318376E-14,
10.));
#26236=CARTESIAN_POINT('Origin',(35.7976661819107,9.54097911787244E-15,
-10.));
#26237=CARTESIAN_POINT('',(204.,-1.28397303707684E-14,-10.));
#26238=CARTESIAN_POINT('Origin',(6.93889390390723E-15,1.21430643318376E-14,
-10.));
#26239=CARTESIAN_POINT('Origin',(6.93889390390723E-15,1.21430643318376E-14,
-10.));
#26240=CARTESIAN_POINT('',(184.50486486776,91.6185289127127,-10.));
#26241=CARTESIAN_POINT('',(184.50486486776,-91.6185289127127,-10.));
#26242=CARTESIAN_POINT('Origin',(71.5953323638214,6.93889390390723E-15,
-10.));
#26243=CARTESIAN_POINT('Origin',(-6.93889390390723E-15,1.21430643318376E-14,
-10.));
#26244=CARTESIAN_POINT('Origin',(210.,0.,0.));
#26245=CARTESIAN_POINT('Origin',(71.5953323638214,6.93889390390723E-15,
-7.));
#26246=CARTESIAN_POINT('',(184.50486486776,-91.6185289127127,-7.));
#26247=CARTESIAN_POINT('',(184.50486486776,-91.6185289127127,-7.));
#26248=CARTESIAN_POINT('',(184.50486486776,91.6185289127127,-7.));
#26249=CARTESIAN_POINT('Origin',(71.5953323638214,6.93889390390723E-15,
-7.));
#26250=CARTESIAN_POINT('',(184.50486486776,91.6185289127127,-7.));
#26251=CARTESIAN_POINT('Origin',(-6.93889390390723E-15,1.21430643318376E-14,
-7.));
#26252=CARTESIAN_POINT('Origin',(-6.93889390390723E-15,1.21430643318376E-14,
-7.));
#26253=CARTESIAN_POINT('Origin',(35.7976661819107,9.54097911787244E-15,
-7.));
#26254=CARTESIAN_POINT('Origin',(35.7976661819107,9.54097911787244E-15,
7.));
#26255=CARTESIAN_POINT('Origin',(6.93889390390723E-15,1.21430643318376E-14,
12.5));
#26256=CARTESIAN_POINT('Ctrl Pts',(203.969311528224,3.53835480166773,3.5327107576923));
#26257=CARTESIAN_POINT('Ctrl Pts',(203.985313878591,2.61589547515511,4.45664385360227));
#26258=CARTESIAN_POINT('Ctrl Pts',(204.,1.32135029102454,5.));
#26259=CARTESIAN_POINT('Ctrl Pts',(204.,1.86713497344704E-14,5.));
#26260=CARTESIAN_POINT('Origin',(6.93889390390723E-15,1.21430643318376E-14,
12.5));
#26261=CARTESIAN_POINT('Ctrl Pts',(204.,1.86713497344704E-14,5.));
#26262=CARTESIAN_POINT('Ctrl Pts',(204.,-1.32135029102454,5.));
#26263=CARTESIAN_POINT('Ctrl Pts',(203.985345962115,-2.61339289425715,4.45784180166547));
#26264=CARTESIAN_POINT('Ctrl Pts',(203.969354900227,-3.535853727891,3.53521405504098));
#26265=CARTESIAN_POINT('Origin',(6.93889390390723E-15,1.21430643318376E-14,
12.5));
#26266=CARTESIAN_POINT('Ctrl Pts',(203.969354900227,-3.535853727891,3.53521405504098));
#26267=CARTESIAN_POINT('Ctrl Pts',(203.95336383834,-4.45831456152485,2.61258630841649));
#26268=CARTESIAN_POINT('Ctrl Pts',(203.938733312599,-4.99930548519226,1.30702665821117));
#26269=CARTESIAN_POINT('Ctrl Pts',(203.938716302406,-4.99999929267631,0.00265955567476928));
#26270=CARTESIAN_POINT('Origin',(6.93889390390723E-15,1.21430643318376E-14,
12.5));
#26271=CARTESIAN_POINT('Ctrl Pts',(203.938716302406,-4.99999929267631,0.00265955567476928));
#26272=CARTESIAN_POINT('Ctrl Pts',(203.938699292213,-5.00069310016037,-1.30170754686164));
#26273=CARTESIAN_POINT('Ctrl Pts',(203.953150206634,-4.47024776275284,-2.59986968375128));
#26274=CARTESIAN_POINT('Ctrl Pts',(203.969329275085,-3.5373316316096,-3.53373526569467));
#26275=CARTESIAN_POINT('Origin',(6.93889390390723E-15,1.21430643318376E-14,
12.5));
#26276=CARTESIAN_POINT('Ctrl Pts',(203.969329275182,-3.53733162599185,-3.53373527131814));
#26277=CARTESIAN_POINT('Ctrl Pts',(203.985508343594,-2.60441549525788,-4.4676008497735));
#26278=CARTESIAN_POINT('Ctrl Pts',(203.99998865724,-1.30698993165052,-4.99953721534887));
#26279=CARTESIAN_POINT('Ctrl Pts',(203.999999994872,-0.0014763518149245,
-4.99999979075699));
#26280=CARTESIAN_POINT('Ctrl Pts',(203.999999996688,-0.0011810813606895,
-4.9999998676999));
#26281=CARTESIAN_POINT('Ctrl Pts',(203.999999997836,-0.000885810883897428,
-4.9999999180906));
#26282=CARTESIAN_POINT('Origin',(6.93889390390723E-15,1.21430643318376E-14,
12.5));
#26283=CARTESIAN_POINT('Ctrl Pts',(203.999999999357,-6.80789583155938E-12,
-4.99999999073248));
#26284=CARTESIAN_POINT('Ctrl Pts',(203.999998107003,1.30462817101094,-4.99997309336906));
#26285=CARTESIAN_POINT('Ctrl Pts',(203.985394513333,2.60961113596895,-4.45966517513484));
#26286=CARTESIAN_POINT('Ctrl Pts',(203.96941989844,3.5321022485035,-3.53896223575733));
#26287=CARTESIAN_POINT('Origin',(6.93889390390723E-15,1.21430643318376E-14,
12.5));
#26288=CARTESIAN_POINT('Ctrl Pts',(203.96941989844,3.5321022485035,-3.53896223575733));
#26289=CARTESIAN_POINT('Ctrl Pts',(203.953438052627,4.45501092726816,-2.61784253956751));
#26290=CARTESIAN_POINT('Ctrl Pts',(203.938749239315,4.99865586979689,-1.32397596744565));
#26291=CARTESIAN_POINT('Ctrl Pts',(203.938716348481,4.99999741338323,-0.00508587858850664));
#26292=CARTESIAN_POINT('Origin',(6.93889390390723E-15,1.21430643318376E-14,
12.5));
#26293=CARTESIAN_POINT('Ctrl Pts',(203.938716348481,4.99999741338354,-0.0050858782837947));
#26294=CARTESIAN_POINT('Ctrl Pts',(203.938683457647,5.00133895697019,1.31380421087806));
#26295=CARTESIAN_POINT('Ctrl Pts',(203.953309177856,4.46081412818035,2.60877766178233));
#26296=CARTESIAN_POINT('Ctrl Pts',(203.969311528224,3.5383548016686,3.53271075769143));
#26297=CARTESIAN_POINT('Ctrl Pts',(-203.999999992307,-0.00177162224218141,
-4.99999968613545));
#26298=CARTESIAN_POINT('Ctrl Pts',(-199.974620125014,-0.00177162224218141,
-4.99999968613545));
#26299=CARTESIAN_POINT('Ctrl Pts',(-204.000011327375,1.30344668978611,-5.00046215692299));
#26300=CARTESIAN_POINT('Ctrl Pts',(-199.974631460081,1.30344668978611,-5.00046215692299));
#26301=CARTESIAN_POINT('Ctrl Pts',(-203.985401744253,2.60919356973881,-4.46008193194718));
#26302=CARTESIAN_POINT('Ctrl Pts',(-199.96002187696,2.60919356973881,-4.46008193194718));
#26303=CARTESIAN_POINT('Ctrl Pts',(-203.953438052627,4.45501092726815,-2.61784253956752));
#26304=CARTESIAN_POINT('Ctrl Pts',(-199.928058185333,4.45501092726815,-2.61784253956752));
#26305=CARTESIAN_POINT('Ctrl Pts',(-203.938749239315,4.99865586979689,-1.32397596744566));
#26306=CARTESIAN_POINT('Ctrl Pts',(-199.913369372021,4.99865586979689,-1.32397596744566));
#26307=CARTESIAN_POINT('Ctrl Pts',(-203.938683457647,5.00133895697019,1.31380421087806));
#26308=CARTESIAN_POINT('Ctrl Pts',(-199.913303590353,5.00133895697019,1.31380421087806));
#26309=CARTESIAN_POINT('Ctrl Pts',(-203.953309177856,4.46081412818036,2.60877766178232));
#26310=CARTESIAN_POINT('Ctrl Pts',(-199.927929310562,4.46081412818036,2.60877766178232));
#26311=CARTESIAN_POINT('Ctrl Pts',(-203.985313878591,2.61589547515512,4.45664385360227));
#26312=CARTESIAN_POINT('Ctrl Pts',(-199.959934011298,2.61589547515512,4.45664385360227));
#26313=CARTESIAN_POINT('Ctrl Pts',(-204.,1.32135029102454,5.));
#26314=CARTESIAN_POINT('Ctrl Pts',(-199.974620132706,1.32135029102454,5.));
#26315=CARTESIAN_POINT('Ctrl Pts',(-204.,1.12757025938492E-14,5.));
#26316=CARTESIAN_POINT('Ctrl Pts',(-199.974620132706,1.12757025938492E-14,
5.));
#26317=CARTESIAN_POINT('',(-199.999999992153,-0.00177162224212464,-4.99999968613545));
#26318=CARTESIAN_POINT('',(-203.999999992307,-0.00177162224212464,-4.99999968613545));
#26319=CARTESIAN_POINT('',(-200.,1.12757025938492E-14,5.));
#26320=CARTESIAN_POINT('Ctrl Pts',(-199.999999992153,-0.00177162224212553,
-4.99999968613545));
#26321=CARTESIAN_POINT('Ctrl Pts',(-200.000003044699,0.342832911795084,
-5.00012178795457));
#26322=CARTESIAN_POINT('Ctrl Pts',(-199.999103488806,0.687139768358673,
-4.96254505217617));
#26323=CARTESIAN_POINT('Ctrl Pts',(-199.995649725478,1.36161627231926,-4.81818525737039));
#26324=CARTESIAN_POINT('Ctrl Pts',(-199.993093266738,1.69191513651859,-4.71126381843881));
#26325=CARTESIAN_POINT('Ctrl Pts',(-199.984265249359,2.57114744328878,-4.32586384969142));
#26326=CARTESIAN_POINT('Ctrl Pts',(-199.976588732641,3.09094216142015,-3.97786286150404));
#26327=CARTESIAN_POINT('Ctrl Pts',(-199.964848438847,3.7566290408418,-3.31559837286709));
#26328=CARTESIAN_POINT('Ctrl Pts',(-199.960791072323,3.96423745731536,-3.06259999377541));
#26329=CARTESIAN_POINT('Ctrl Pts',(-199.953200858042,4.33028256236115,-2.51482260163278));
#26330=CARTESIAN_POINT('Ctrl Pts',(-199.94970024374,4.48703860433044,-2.22128115603191));
#26331=CARTESIAN_POINT('Ctrl Pts',(-199.941243543139,4.85350328037375,-1.33869041380516));
#26332=CARTESIAN_POINT('Ctrl Pts',(-199.937819060768,4.98684858575005,-0.719094610949247));
#26333=CARTESIAN_POINT('Ctrl Pts',(-199.937186821031,5.01213494883686,0.572498875379037));
#26334=CARTESIAN_POINT('Ctrl Pts',(-199.940397897686,4.88659419116962,1.19429563481081));
#26335=CARTESIAN_POINT('Ctrl Pts',(-199.950579947465,4.45185250038562,2.36075809964606));
#26336=CARTESIAN_POINT('Ctrl Pts',(-199.9584705221,4.10050445672718,2.93508260604331));
#26337=CARTESIAN_POINT('Ctrl Pts',(-199.96867594025,3.54121851280074,3.53348074247459));
#26338=CARTESIAN_POINT('Ctrl Pts',(-199.970646802731,3.42846001602563,3.64281433950469));
#26339=CARTESIAN_POINT('Ctrl Pts',(-199.980072705603,2.85908134037781,4.1438810712431));
#26340=CARTESIAN_POINT('Ctrl Pts',(-199.987155864494,2.33527138703284,4.45694173085698));
#26341=CARTESIAN_POINT('Ctrl Pts',(-199.997153136931,1.20768836931978,4.88593625759029));
#26342=CARTESIAN_POINT('Ctrl Pts',(-200.,0.605263673202607,5.));
#26343=CARTESIAN_POINT('Ctrl Pts',(-200.,1.13797860024079E-14,5.));
#26344=CARTESIAN_POINT('',(-204.,1.12757025938492E-14,5.));
#26345=CARTESIAN_POINT('Origin',(175.75628980623,72.1784357931688,12.5));
#26346=CARTESIAN_POINT('',(181.394623471171,63.9195500642836,-7.5));
#26347=CARTESIAN_POINT('',(185.006620848663,75.9773008349145,-7.5));
#26348=CARTESIAN_POINT('Origin',(175.75628980623,72.1784357931688,-7.5));
#26349=CARTESIAN_POINT('',(181.394623471171,63.9195500642836,7.5));
#26350=CARTESIAN_POINT('',(181.394623471171,63.9195500642836,7.5));
#26351=CARTESIAN_POINT('',(185.006620848663,75.9773008349145,7.5));
#26352=CARTESIAN_POINT('Origin',(175.75628980623,72.1784357931688,7.5));
#26353=CARTESIAN_POINT('',(185.006620848663,75.9773008349145,12.5));
#26354=CARTESIAN_POINT('Origin',(175.75628980623,-72.1784357931688,7.5));
#26355=CARTESIAN_POINT('',(185.006620848663,-75.9773008349145,-7.5));
#26356=CARTESIAN_POINT('',(181.394623471171,-63.9195500642836,-7.5));
#26357=CARTESIAN_POINT('Origin',(175.75628980623,-72.1784357931688,-7.5));
#26358=CARTESIAN_POINT('',(185.006620848663,-75.9773008349145,7.5));
#26359=CARTESIAN_POINT('',(185.006620848663,-75.9773008349145,12.5));
#26360=CARTESIAN_POINT('',(181.394623471171,-63.9195500642836,7.5));
#26361=CARTESIAN_POINT('Origin',(175.75628980623,-72.1784357931688,7.5));
#26362=CARTESIAN_POINT('',(181.394623471171,-63.9195500642836,7.5));
#26363=CARTESIAN_POINT('Ctrl Pts',(204.,2.16840434497101E-16,5.));
#26364=CARTESIAN_POINT('Ctrl Pts',(199.974623012481,2.16840434497101E-16,
5.));
#26365=CARTESIAN_POINT('Ctrl Pts',(204.,-1.32135029102454,5.));
#26366=CARTESIAN_POINT('Ctrl Pts',(199.974623012481,-1.32135029102454,5.));
#26367=CARTESIAN_POINT('Ctrl Pts',(203.985345962115,-2.61339289425715,4.45784180166547));
#26368=CARTESIAN_POINT('Ctrl Pts',(199.959968974597,-2.61339289425715,4.45784180166547));
#26369=CARTESIAN_POINT('Ctrl Pts',(203.95336383834,-4.45831456152485,2.61258630841649));
#26370=CARTESIAN_POINT('Ctrl Pts',(199.927986850821,-4.45831456152485,2.61258630841649));
#26371=CARTESIAN_POINT('Ctrl Pts',(203.938733312599,-4.99930548519226,1.30702665821117));
#26372=CARTESIAN_POINT('Ctrl Pts',(199.91335632508,-4.99930548519226,1.30702665821117));
#26373=CARTESIAN_POINT('Ctrl Pts',(203.938699292213,-5.00069310016037,-1.30170754686164));
#26374=CARTESIAN_POINT('Ctrl Pts',(199.913322304694,-5.00069310016037,-1.30170754686164));
#26375=CARTESIAN_POINT('Ctrl Pts',(203.953150206634,-4.47024776275284,-2.59986968375128));
#26376=CARTESIAN_POINT('Ctrl Pts',(199.927773219115,-4.47024776275284,-2.59986968375128));
#26377=CARTESIAN_POINT('Ctrl Pts',(203.985508343536,-2.60441550046636,-4.46760084763805));
#26378=CARTESIAN_POINT('Ctrl Pts',(199.960131356017,-2.60441550046636,-4.46760084763805));
#26379=CARTESIAN_POINT('Ctrl Pts',(203.99998865724,-1.3069899342704,-4.99953721534794));
#26380=CARTESIAN_POINT('Ctrl Pts',(199.974611669721,-1.3069899342704,-4.99953721534794));
#26381=CARTESIAN_POINT('Ctrl Pts',(204.000000269508,0.03014770113918,-5.00001099593281));
#26382=CARTESIAN_POINT('Ctrl Pts',(199.974623281989,0.03014770113918,-5.00001099593281));
#26383=CARTESIAN_POINT('Ctrl Pts',(203.999991802598,0.0620673406330946,
-4.99969885211784));
#26384=CARTESIAN_POINT('Ctrl Pts',(199.974614815079,0.0620673406330946,
-4.99969885211784));
#26385=CARTESIAN_POINT('Ctrl Pts',(203.999974785344,0.0939816892981964,
-4.99906559628474));
#26386=CARTESIAN_POINT('Ctrl Pts',(199.974597797825,0.0939816892981964,
-4.99906559628474));
#26387=CARTESIAN_POINT('',(199.999999992153,-0.0017716222421091,-4.99999968613545));
#26388=CARTESIAN_POINT('',(203.999999992307,-0.0017716222421091,-4.99999968613545));
#26389=CARTESIAN_POINT('',(200.,2.16840434497101E-16,5.));
#26390=CARTESIAN_POINT('Ctrl Pts',(200.,2.16840434497101E-16,5.));
#26391=CARTESIAN_POINT('Ctrl Pts',(200.,-0.106689085431466,5.));
#26392=CARTESIAN_POINT('Ctrl Pts',(199.999913765457,-0.212770994842209,
4.99646994038258));
#26393=CARTESIAN_POINT('Ctrl Pts',(199.999745448447,-0.318263257811292,
4.98955065372514));
#26394=CARTESIAN_POINT('Ctrl Pts',(199.999569044592,-0.428823930404872,
4.98229892772));
#26395=CARTESIAN_POINT('Ctrl Pts',(199.999302473722,-0.538737440023033,
4.97132466138716));
#26396=CARTESIAN_POINT('Ctrl Pts',(199.998948825096,-0.64802295579962,4.95672957226209));
#26397=CARTESIAN_POINT('Ctrl Pts',(199.998595176469,-0.757308471576208,
4.94213448313703));
#26398=CARTESIAN_POINT('Ctrl Pts',(199.99815442921,-0.86596652308077,4.92391831426076));
#26399=CARTESIAN_POINT('Ctrl Pts',(199.997628259871,-0.974007405778188,
4.90212506063419));
#26400=CARTESIAN_POINT('Ctrl Pts',(199.99714301239,-1.07364560643664,4.88202673744735));
#26401=CARTESIAN_POINT('Ctrl Pts',(199.996583375234,-1.17308267575688,4.85881220605306));
#26402=CARTESIAN_POINT('Ctrl Pts',(199.995954265594,-1.2719366915673,4.83253690787655));
#26403=CARTESIAN_POINT('Ctrl Pts',(199.995322421172,-1.37122043236585,4.80614738922954));
#26404=CARTESIAN_POINT('Ctrl Pts',(199.994620514446,-1.46991557653475,4.77667056294847));
#26405=CARTESIAN_POINT('Ctrl Pts',(199.993854778568,-1.56764391846616,4.74421450831223));
#26406=CARTESIAN_POINT('Ctrl Pts',(199.993085898829,-1.66577350100801,4.71162519973023));
#26407=CARTESIAN_POINT('Ctrl Pts',(199.99225268186,-1.7629278505394,4.67603232253121));
#26408=CARTESIAN_POINT('Ctrl Pts',(199.991362450625,-1.85873994433746,4.6375952416386));
#26409=CARTESIAN_POINT('Ctrl Pts',(199.991194313089,-1.87683592740531,4.63033564906069));
#26410=CARTESIAN_POINT('Ctrl Pts',(199.991024144215,-1.89488408714042,4.62297473700675));
#26411=CARTESIAN_POINT('Ctrl Pts',(199.990851996581,-1.9128820355165,4.61551376963032));
#26412=CARTESIAN_POINT('Ctrl Pts',(199.989904874678,-2.0119031527102,4.57446501732134));
#26413=CARTESIAN_POINT('Ctrl Pts',(199.988899457036,-2.10927871151272,4.5304446155066));
#26414=CARTESIAN_POINT('Ctrl Pts',(199.987843468119,-2.20502888607493,4.48349555287741));
#26415=CARTESIAN_POINT('Ctrl Pts',(199.986757493131,-2.30349800157137,4.43521331536066));
#26416=CARTESIAN_POINT('Ctrl Pts',(199.985618017166,-2.40024873740821,4.38383369997872));
#26417=CARTESIAN_POINT('Ctrl Pts',(199.984432539852,-2.49528004230067,4.32935098461817));
#26418=CARTESIAN_POINT('Ctrl Pts',(199.983247062538,-2.59031134719313,4.27486826925761));
#26419=CARTESIAN_POINT('Ctrl Pts',(199.982015562515,-2.68362377963686,4.21728220600999));
#26420=CARTESIAN_POINT('Ctrl Pts',(199.980744946283,-2.7751848100423,4.15653780080854));
#26421=CARTESIAN_POINT('Ctrl Pts',(199.979687255077,-2.85140239185876,4.1059727115688));
#26422=CARTESIAN_POINT('Ctrl Pts',(199.97860051674,-2.92654667296149,4.05311678026368));
#26423=CARTESIAN_POINT('Ctrl Pts',(199.977494181696,-3.00027821604381,3.99812698249647));
#26424=CARTESIAN_POINT('Ctrl Pts',(199.976393937544,-3.07360383248166,3.94343992929629));
#26425=CARTESIAN_POINT('Ctrl Pts',(199.975274327858,-3.14553183008494,3.88664264849037));
#26426=CARTESIAN_POINT('Ctrl Pts',(199.974145117418,-3.21575710331105,3.82793200561578));
#26427=CARTESIAN_POINT('Ctrl Pts',(199.973025477997,-3.28538715766477,3.76971898533551));
#26428=CARTESIAN_POINT('Ctrl Pts',(199.971896415521,-3.35334289802745,3.70962515179665));
#26429=CARTESIAN_POINT('Ctrl Pts',(199.970767675607,-3.4193606338094,3.64788081938912));
#26430=CARTESIAN_POINT('Ctrl Pts',(199.970092075891,-3.45887510736828,3.61092416279631));
#26431=CARTESIAN_POINT('Ctrl Pts',(199.969416594983,-3.49769595480584,3.57337692877078));
#26432=CARTESIAN_POINT('Ctrl Pts',(199.968743327175,-3.53577320405375,3.53529459154323));
#26433=CARTESIAN_POINT('Ctrl Pts',(199.968742852571,-3.53580004566718,3.53526774634316));
#26434=CARTESIAN_POINT('Ctrl Pts',(199.968742377966,-3.53582688694626,3.53524090084241));
#26435=CARTESIAN_POINT('Ctrl Pts',(199.96874190336,-3.535853727891,3.53521405504098));
#26436=CARTESIAN_POINT('Ctrl Pts',(199.967444306764,-3.60923812432215,3.46181638020426));
#26437=CARTESIAN_POINT('Ctrl Pts',(199.96615206232,-3.68005108078868,3.38615882914448));
#26438=CARTESIAN_POINT('Ctrl Pts',(199.96487158156,-3.74836710179276,3.30830569203447));
#26439=CARTESIAN_POINT('Ctrl Pts',(199.963578976184,-3.81732999356935,3.22971537910238));
#26440=CARTESIAN_POINT('Ctrl Pts',(199.962298340419,-3.88374870865775,3.14888724771301));
#26441=CARTESIAN_POINT('Ctrl Pts',(199.961036490357,-3.94766064633092,3.06585149887276));
#26442=CARTESIAN_POINT('Ctrl Pts',(199.959767630887,-4.01192760623837,2.98235449759437));
#26443=CARTESIAN_POINT('Ctrl Pts',(199.958517747431,-4.07366014492571,2.8966247993813));
#26444=CARTESIAN_POINT('Ctrl Pts',(199.957294270602,-4.13285266907493,2.80866409496906));
#26445=CARTESIAN_POINT('Ctrl Pts',(199.95715658911,-4.1395137801211,2.79876561491249));
#26446=CARTESIAN_POINT('Ctrl Pts',(199.95701924272,-4.14614267734788,2.78883885657405));
#26447=CARTESIAN_POINT('Ctrl Pts',(199.956882242583,-4.15273931588746,2.77888380377105));
#26448=CARTESIAN_POINT('Ctrl Pts',(199.955449809748,-4.22171181380409,2.67479672144946));
#26449=CARTESIAN_POINT('Ctrl Pts',(199.954061738709,-4.28685552062367,2.56806446766188));
#26450=CARTESIAN_POINT('Ctrl Pts',(199.952733419607,-4.34795058538834,2.45918048333498));
#26451=CARTESIAN_POINT('Ctrl Pts',(199.951403408826,-4.40912345767029,2.35015782999244));
#26452=CARTESIAN_POINT('Ctrl Pts',(199.950133324122,-4.46623711429618,2.23897860351396));
#26453=CARTESIAN_POINT('Ctrl Pts',(199.9489378304,-4.51911833478099,2.12615944454101));
#26454=CARTESIAN_POINT('Ctrl Pts',(199.948189148404,-4.55223537839354,2.05550606374186));
#26455=CARTESIAN_POINT('Ctrl Pts',(199.947469703677,-4.58369344773626,1.98420990101436));
#26456=CARTESIAN_POINT('Ctrl Pts',(199.946782884472,-4.61346010600003,1.91240038834254));
#26457=CARTESIAN_POINT('Ctrl Pts',(199.945244027409,-4.68015397830596,1.75150713569573));
#26458=CARTESIAN_POINT('Ctrl Pts',(199.943856293168,-4.73891591400558,1.58668724722363));
#26459=CARTESIAN_POINT('Ctrl Pts',(199.942652291709,-4.78917781231223,1.41890179219067));
#26460=CARTESIAN_POINT('Ctrl Pts',(199.941603883869,-4.83294434421902,1.27279932255469));
#26461=CARTESIAN_POINT('Ctrl Pts',(199.940694808887,-4.87026604656124,1.12444934574699));
#26462=CARTESIAN_POINT('Ctrl Pts',(199.93994672643,-4.90078596068217,0.97451290256118));
#26463=CARTESIAN_POINT('Ctrl Pts',(199.939427256788,-4.92197903732505,0.870396799239052));
#26464=CARTESIAN_POINT('Ctrl Pts',(199.938988357527,-4.93977769850371,0.766104978382168));
#26465=CARTESIAN_POINT('Ctrl Pts',(199.938631378381,-4.95419932372897,0.661646608836728));
#26466=CARTESIAN_POINT('Ctrl Pts',(199.938257638965,-4.96929804824499,0.552283889966628));
#26467=CARTESIAN_POINT('Ctrl Pts',(199.937973662438,-4.98069584574989,0.442738086255646));
#26468=CARTESIAN_POINT('Ctrl Pts',(199.937782272973,-4.98835300268517,0.333005356104372));
#26469=CARTESIAN_POINT('Ctrl Pts',(199.937602385329,-4.99554999187858,0.229867170517087));
#26470=CARTESIAN_POINT('Ctrl Pts',(199.937504286432,-4.9994420905526,0.126563270571131));
#26471=CARTESIAN_POINT('Ctrl Pts',(199.93749163394,-4.99994428099095,0.0230865138943863));
#26472=CARTESIAN_POINT('Ctrl Pts',(199.937490824953,-4.999976390507,0.0164703214593889));
#26473=CARTESIAN_POINT('Ctrl Pts',(199.937490365772,-4.99999462369657,0.00985342259099019));
#26474=CARTESIAN_POINT('Ctrl Pts',(199.937490257555,-4.99999895100585,0.00323581564284581));
#26475=CARTESIAN_POINT('Ctrl Pts',(199.937490254414,-4.99999907661166,0.00304373094603564));
#26476=CARTESIAN_POINT('Ctrl Pts',(199.937490251566,-4.99999919050222,0.00285164428893937));
#26477=CARTESIAN_POINT('Ctrl Pts',(199.937490249012,-4.99999929267631,0.00265955567476706));
#26478=CARTESIAN_POINT('Ctrl Pts',(199.937489018394,-5.00004851957456,-0.0898876539113899));
#26479=CARTESIAN_POINT('Ctrl Pts',(199.937555311217,-4.99741975626774,-0.182864304129975));
#26480=CARTESIAN_POINT('Ctrl Pts',(199.937688351935,-4.99210548145091,-0.275917349116757));
#26481=CARTESIAN_POINT('Ctrl Pts',(199.937822179922,-4.98675975940393,-0.369521035653615));
#26482=CARTESIAN_POINT('Ctrl Pts',(199.938023535793,-4.97869670329359,-0.463201602984161));
#26483=CARTESIAN_POINT('Ctrl Pts',(199.938290146696,-4.96796164010122,-0.556598752708217));
#26484=CARTESIAN_POINT('Ctrl Pts',(199.938559009805,-4.95713589206307,-0.650784878330061));
#26485=CARTESIAN_POINT('Ctrl Pts',(199.938894221282,-4.94359288463427,-0.744682328172369));
#26486=CARTESIAN_POINT('Ctrl Pts',(199.939292143069,-4.92743182557626,-0.837927234917629));
#26487=CARTESIAN_POINT('Ctrl Pts',(199.939485856061,-4.9195644325493,-0.883319948754859));
#26488=CARTESIAN_POINT('Ctrl Pts',(199.939694412193,-4.91107738214136,-0.928558146494761));
#26489=CARTESIAN_POINT('Ctrl Pts',(199.939917296751,-4.90198647168346,-0.97360081736077));
#26490=CARTESIAN_POINT('Ctrl Pts',(199.940432998254,-4.88095228143802,-1.07781877358698));
#26491=CARTESIAN_POINT('Ctrl Pts',(199.941025461062,-4.85667571130338,-1.18106633062347));
#26492=CARTESIAN_POINT('Ctrl Pts',(199.941688795583,-4.82922287471879,-1.28335964226709));
#26493=CARTESIAN_POINT('Ctrl Pts',(199.942377799029,-4.80070770109351,-1.3896113781573));
#26494=CARTESIAN_POINT('Ctrl Pts',(199.943143277803,-4.76876581556843,-1.49483421604507));
#26495=CARTESIAN_POINT('Ctrl Pts',(199.943979937156,-4.73341334147567,-1.59903492791101));
#26496=CARTESIAN_POINT('Ctrl Pts',(199.944816596509,-4.6980608673829,-1.70323563977696));
#26497=CARTESIAN_POINT('Ctrl Pts',(199.945724457359,-4.65929760501924,-1.80641482603871));
#26498=CARTESIAN_POINT('Ctrl Pts',(199.946699239106,-4.6170838617614,-1.908558894064));
#26499=CARTESIAN_POINT('Ctrl Pts',(199.947580381323,-4.57892525707422,-2.00089079386994));
#26500=CARTESIAN_POINT('Ctrl Pts',(199.948516093717,-4.53794998813828,-2.09234828060927));
#26501=CARTESIAN_POINT('Ctrl Pts',(199.949497749981,-4.49428712854347,-2.18256058459083));
#26502=CARTESIAN_POINT('Ctrl Pts',(199.950476582438,-4.45074986841002,-2.27251338617393));
#26503=CARTESIAN_POINT('Ctrl Pts',(199.951501077809,-4.40454064733321,-2.36122769950356));
#26504=CARTESIAN_POINT('Ctrl Pts',(199.952561949357,-4.35583435975879,-2.44835766561793));
#26505=CARTESIAN_POINT('Ctrl Pts',(199.953616658299,-4.30741100717498,-2.53498149346203));
#26506=CARTESIAN_POINT('Ctrl Pts',(199.954707305024,-4.25651975128412,-2.6200389191733));
#26507=CARTESIAN_POINT('Ctrl Pts',(199.955824291131,-4.20337569014082,-2.7032180367477));
#26508=CARTESIAN_POINT('Ctrl Pts',(199.956150084129,-4.18787508284152,-2.72747901359602));
#26509=CARTESIAN_POINT('Ctrl Pts',(199.956478115705,-4.17218309328504,-2.75158040235868));
#26510=CARTESIAN_POINT('Ctrl Pts',(199.956808143247,-4.15630571119065,-2.77551499023631));
#26511=CARTESIAN_POINT('Ctrl Pts',(199.958041623657,-4.09696387664856,-2.86497069176347));
#26512=CARTESIAN_POINT('Ctrl Pts',(199.959307171522,-4.03482709407707,-2.95241426289202));
#26513=CARTESIAN_POINT('Ctrl Pts',(199.96059705484,-3.96986498972616,-3.03782589478993));
#26514=CARTESIAN_POINT('Ctrl Pts',(199.961908169114,-3.90383363549083,-3.12464336749992));
#26515=CARTESIAN_POINT('Ctrl Pts',(199.963244443955,-3.83488312168669,-3.2093620691675));
#26516=CARTESIAN_POINT('Ctrl Pts',(199.964598170151,-3.76293631072323,-3.29192868462007));
#26517=CARTESIAN_POINT('Ctrl Pts',(199.965951896348,-3.69098949975976,-3.37449530007264));
#26518=CARTESIAN_POINT('Ctrl Pts',(199.967323092874,-3.6160462267238,-3.45491039126157));
#26519=CARTESIAN_POINT('Ctrl Pts',(199.968704181971,-3.5379864023958,-3.5330797025401));
#26520=CARTESIAN_POINT('Ctrl Pts',(199.968708043156,-3.53776816634513,-3.53329824468933));
#26521=CARTESIAN_POINT('Ctrl Pts',(199.968711904499,-3.53754990941597,-3.53351676574182));
#26522=CARTESIAN_POINT('Ctrl Pts',(199.968715766001,-3.5373316316096,-3.53373526569467));
#26523=CARTESIAN_POINT('Ctrl Pts',(199.970460080863,-3.43873133816247,-3.63243590699128));
#26524=CARTESIAN_POINT('Ctrl Pts',(199.972198401154,-3.3362985501167,-3.7264135444678));
#26525=CARTESIAN_POINT('Ctrl Pts',(199.97390904525,-3.23039259847156,-3.81566238109671));
#26526=CARTESIAN_POINT('Ctrl Pts',(199.97565820908,-3.12210189066793,-3.9069208943253));
#26527=CARTESIAN_POINT('Ctrl Pts',(199.977378458043,-3.0101793631941,-3.993235586349));
#26528=CARTESIAN_POINT('Ctrl Pts',(199.979046584675,-2.89497000257252,-4.07456267017766));
#26529=CARTESIAN_POINT('Ctrl Pts',(199.979597895658,-2.85689364512564,-4.10144103402992));
#26530=CARTESIAN_POINT('Ctrl Pts',(199.980143511741,-2.81845799249297,-4.12777428808935));
#26531=CARTESIAN_POINT('Ctrl Pts',(199.980682588089,-2.779674729519,-4.15355987795212));
#26532=CARTESIAN_POINT('Ctrl Pts',(199.98193608989,-2.68949290247773,-4.21351851543761));
#26533=CARTESIAN_POINT('Ctrl Pts',(199.983159605131,-2.59702475383697,-4.27078090386246));
#26534=CARTESIAN_POINT('Ctrl Pts',(199.984340873962,-2.5026016568129,-4.32510605962663));
#26535=CARTESIAN_POINT('Ctrl Pts',(199.985531674906,-2.40741662352963,-4.37986958595127));
#26536=CARTESIAN_POINT('Ctrl Pts',(199.986679526008,-2.31024539867246,-4.43164800699807));
#26537=CARTESIAN_POINT('Ctrl Pts',(199.987772232853,-2.21145908473947,-4.48023721650249));
#26538=CARTESIAN_POINT('Ctrl Pts',(199.988854707941,-2.11359777432304,-4.52837145215608));
#26539=CARTESIAN_POINT('Ctrl Pts',(199.989883049636,-2.01415200784204,-4.57337579928167));
#26540=CARTESIAN_POINT('Ctrl Pts',(199.990846026127,-1.91350614164553,-4.61509643176659));
#26541=CARTESIAN_POINT('Ctrl Pts',(199.991792578593,-1.81457683876425,-4.65610549893921));
#26542=CARTESIAN_POINT('Ctrl Pts',(199.992673774464,-1.71473372931631,-4.69384912859574));
#26543=CARTESIAN_POINT('Ctrl Pts',(199.993486393832,-1.61399492664038,-4.72837579232869));
#26544=CARTESIAN_POINT('Ctrl Pts',(199.994324637516,-1.51007952850957,-4.76399118493446));
#26545=CARTESIAN_POINT('Ctrl Pts',(199.995089935849,-1.40521060202274,-4.79618398138844));
#26546=CARTESIAN_POINT('Ctrl Pts',(199.995777839267,-1.29938616025944,-4.82495380140898));
#26547=CARTESIAN_POINT('Ctrl Pts',(199.996465742685,-1.19356171849615,-4.85372362142952));
#26548=CARTESIAN_POINT('Ctrl Pts',(199.997076272279,-1.08678118101417,-4.87907068709132));
#26549=CARTESIAN_POINT('Ctrl Pts',(199.997603740834,-0.979029072207799,
-4.90093718328589));
#26550=CARTESIAN_POINT('Ctrl Pts',(199.998041002663,-0.889704535897929,
-4.91906411049815));
#26551=CARTESIAN_POINT('Ctrl Pts',(199.998421910603,-0.79950470998423,-4.93483341824134));
#26552=CARTESIAN_POINT('Ctrl Pts',(199.998743013132,-0.708780352003267,
-4.94811276998379));
#26553=CARTESIAN_POINT('Ctrl Pts',(199.999062276332,-0.618575678342215,
-4.96131605537501));
#26554=CARTESIAN_POINT('Ctrl Pts',(199.999322402601,-0.527852889977945,
-4.97205769316921));
#26555=CARTESIAN_POINT('Ctrl Pts',(199.999521129845,-0.436966717445114,
-4.98025786975492));
#26556=CARTESIAN_POINT('Ctrl Pts',(199.99971810453,-0.346882062393027,-4.98838572967578));
#26557=CARTESIAN_POINT('Ctrl Pts',(199.999854746094,-0.256637304781016,
-4.99401669744085));
#26558=CARTESIAN_POINT('Ctrl Pts',(199.999930165345,-0.166581446645463,
-4.9971239797482));
#26559=CARTESIAN_POINT('Ctrl Pts',(199.99997625447,-0.11154780929047,-4.99902285730267));
#26560=CARTESIAN_POINT('Ctrl Pts',(199.999999506613,-0.0565847596115855,
-4.99998026449957));
#26561=CARTESIAN_POINT('Ctrl Pts',(199.999999992153,-0.00177162224210914,
-4.99999968613545));
#26562=CARTESIAN_POINT('',(204.,2.16840434497101E-16,5.));
#26563=CARTESIAN_POINT('Origin',(-198.037532067764,0.,-7.5));
#26564=CARTESIAN_POINT('',(-198.037532067764,-27.9488084273619,-7.5));
#26565=CARTESIAN_POINT('',(-198.037532067764,27.948808427362,-7.5));
#26566=CARTESIAN_POINT('Origin',(-198.037532067764,0.,-7.5));
#26567=CARTESIAN_POINT('',(-198.037532067764,-27.948808427362,7.5));
#26568=CARTESIAN_POINT('',(-198.037532067764,-27.9488084273619,-7.5));
#26569=CARTESIAN_POINT('',(-198.037532067764,27.9488084273619,7.5));
#26570=CARTESIAN_POINT('Origin',(-198.037532067764,0.,7.5));
#26571=CARTESIAN_POINT('',(-198.037532067764,27.9488084273619,-7.5));
#26572=CARTESIAN_POINT('Origin',(0.,0.,-78.2106781186548));
#26573=CARTESIAN_POINT('',(2.47860448411075,17.2857000454522,-7.50000000000001));
#26574=CARTESIAN_POINT('',(-2.0402937480676,17.3428979029341,-7.50000000000001));
#26575=CARTESIAN_POINT('Origin',(0.,0.,-7.50000000000001));
#26576=CARTESIAN_POINT('',(-2.0402937480676,17.3428979029341,15.));
#26577=CARTESIAN_POINT('',(-2.0402937480676,17.3428979029341,-78.2106781186548));
#26578=CARTESIAN_POINT('',(2.47860448411075,17.2857000454522,15.));
#26579=CARTESIAN_POINT('Origin',(0.,0.,15.));
#26580=CARTESIAN_POINT('',(2.47860448411075,17.2857000454522,-78.2106781186548));
#26581=CARTESIAN_POINT('Origin',(0.745999527119512,1.21430643318376E-14,
-78.2106781186548));
#26582=CARTESIAN_POINT('',(23.3816321893336,-10.6126402926561,7.5));
#26583=CARTESIAN_POINT('',(25.6668951325528,1.98719959316974,7.5));
#26584=CARTESIAN_POINT('Origin',(0.745999527119512,1.21430643318376E-14,
7.5));
#26585=CARTESIAN_POINT('',(25.6668951325528,1.98719959316974,15.));
#26586=CARTESIAN_POINT('',(25.6668951325528,1.98719959316974,-78.2106781186548));
#26587=CARTESIAN_POINT('',(23.3816321893336,-10.6126402926561,15.));
#26588=CARTESIAN_POINT('Origin',(0.745999527119512,1.21430643318376E-14,
15.));
#26589=CARTESIAN_POINT('',(23.3816321893336,-10.6126402926561,-78.2106781186548));
#26590=CARTESIAN_POINT('Origin',(6.93889390390723E-15,1.21430643318376E-14,
12.5));
#26591=CARTESIAN_POINT('',(204.,-1.28397303707684E-14,-12.5));
#26592=CARTESIAN_POINT('Origin',(6.93889390390723E-15,1.21430643318376E-14,
-12.5));
#26593=CARTESIAN_POINT('',(204.,-1.28397303707684E-14,12.5));
#26594=CARTESIAN_POINT('',(204.,-1.28397303707684E-14,12.5));
#26595=CARTESIAN_POINT('',(204.,-1.28397303707684E-14,12.5));
#26596=CARTESIAN_POINT('Origin',(6.93889390390723E-15,1.21430643318376E-14,
12.5));
#26597=CARTESIAN_POINT('Origin',(6.93889390390723E-15,1.21430643318376E-14,
12.5));
#26598=CARTESIAN_POINT('',(200.,-1.23498716511094E-14,12.5));
#26599=CARTESIAN_POINT('Origin',(6.93889390390723E-15,1.21430643318376E-14,
12.5));
#26600=CARTESIAN_POINT('',(200.,-1.23498716511094E-14,12.5));
#26601=CARTESIAN_POINT('',(200.,-1.22464679914735E-14,-4.99999998173599));
#26602=CARTESIAN_POINT('Ctrl Pts',(200.,-1.40355392239111E-14,-4.99999998173599));
#26603=CARTESIAN_POINT('Ctrl Pts',(200.,-0.00059053984960231,-4.99999999390701));
#26604=CARTESIAN_POINT('Ctrl Pts',(199.999999997384,-0.00118108060876073,
-4.99999989537881));
#26605=CARTESIAN_POINT('Ctrl Pts',(199.999999992153,-0.00177162224210903,
-4.99999968613545));
#26606=CARTESIAN_POINT('',(200.,-1.23498716511094E-14,-12.5));
#26607=CARTESIAN_POINT('',(200.,-1.23498716511094E-14,12.5));
#26608=CARTESIAN_POINT('Origin',(6.93889390390723E-15,1.21430643318376E-14,
-12.5));
#26609=CARTESIAN_POINT('Ctrl Pts',(200.,4.16333634234434E-16,5.));
#26610=CARTESIAN_POINT('Ctrl Pts',(200.,0.605263673276849,5.));
#26611=CARTESIAN_POINT('Ctrl Pts',(199.997153136931,1.20768836943757,4.88593625756298));
#26612=CARTESIAN_POINT('Ctrl Pts',(199.98715586449,2.33527138738033,4.45694173064992));
#26613=CARTESIAN_POINT('Ctrl Pts',(199.980072705597,2.85908134082911,4.14388107086821));
#26614=CARTESIAN_POINT('Ctrl Pts',(199.970646802724,3.42846001642483,3.64281433909067));
#26615=CARTESIAN_POINT('Ctrl Pts',(199.968675940244,3.54121851313504,3.53348074213681));
#26616=CARTESIAN_POINT('Ctrl Pts',(199.958470522096,4.10050445692498,2.93508260589754));
#26617=CARTESIAN_POINT('Ctrl Pts',(199.950579947462,4.45185250050671,2.36075809949633));
#26618=CARTESIAN_POINT('Ctrl Pts',(199.940397897687,4.886594191151,1.19429563484653));
#26619=CARTESIAN_POINT('Ctrl Pts',(199.937186821031,5.01213494884488,0.572498875413951));
#26620=CARTESIAN_POINT('Ctrl Pts',(199.937819060768,4.98684858574211,-0.719094611003917));
#26621=CARTESIAN_POINT('Ctrl Pts',(199.94124354314,4.85350328035862,-1.33869041386019));
#26622=CARTESIAN_POINT('Ctrl Pts',(199.949700243741,4.48703860430459,-2.22128115608432));
#26623=CARTESIAN_POINT('Ctrl Pts',(199.953200858042,4.33028256233193,-2.51482260168344));
#26624=CARTESIAN_POINT('Ctrl Pts',(199.960791072323,3.96423745728102,-3.06259999381995));
#26625=CARTESIAN_POINT('Ctrl Pts',(199.964848438847,3.75662904080501,-3.31559837290915));
#26626=CARTESIAN_POINT('Ctrl Pts',(199.976588732642,3.09094216137304,-3.97786286154054));
#26627=CARTESIAN_POINT('Ctrl Pts',(199.98426524936,2.57114744323512,-4.32586384972337));
#26628=CARTESIAN_POINT('Ctrl Pts',(199.993093266739,1.69191513646751,-4.71126381845647));
#26629=CARTESIAN_POINT('Ctrl Pts',(199.995649725478,1.36161627227762,-4.81818525738156));
#26630=CARTESIAN_POINT('Ctrl Pts',(199.999100531766,0.687717241141568,-4.96242145431402));
#26631=CARTESIAN_POINT('Ctrl Pts',(200.,0.344012953281906,-4.99999289163375));
#26632=CARTESIAN_POINT('Ctrl Pts',(200.,-1.42247325030098E-14,-4.99999998173599));
#26633=CARTESIAN_POINT('Ctrl Pts',(-200.,1.12757025938492E-14,5.));
#26634=CARTESIAN_POINT('Ctrl Pts',(-200.,-0.106689084767584,5.));
#26635=CARTESIAN_POINT('Ctrl Pts',(-199.999913765458,-0.212770993513047,
4.99646994042657));
#26636=CARTESIAN_POINT('Ctrl Pts',(-199.99974544845,-0.318263255820032,
4.98955065385575));
#26637=CARTESIAN_POINT('Ctrl Pts',(-199.999569044596,-0.42882392875795,
4.98229892787329));
#26638=CARTESIAN_POINT('Ctrl Pts',(-199.999302473726,-0.538737438711796,
4.97132466154013));
#26639=CARTESIAN_POINT('Ctrl Pts',(-199.998948825099,-0.648022954821224,
4.95672957239276));
#26640=CARTESIAN_POINT('Ctrl Pts',(-199.998595176472,-0.757308470930653,
4.94213448324538));
#26641=CARTESIAN_POINT('Ctrl Pts',(-199.998154429211,-0.865966522765234,
4.9239183143248));
#26642=CARTESIAN_POINT('Ctrl Pts',(-199.997628259871,-0.97400740579531,
4.90212506063074));
#26643=CARTESIAN_POINT('Ctrl Pts',(-199.997143012391,-1.07364560623553,
4.88202673748756));
#26644=CARTESIAN_POINT('Ctrl Pts',(-199.996583375236,-1.17308267533976,
4.85881220615028));
#26645=CARTESIAN_POINT('Ctrl Pts',(-199.995954265598,-1.27193669093702,
4.83253690804408));
#26646=CARTESIAN_POINT('Ctrl Pts',(-199.995322421178,-1.37122043151843,
4.8061473894685));
#26647=CARTESIAN_POINT('Ctrl Pts',(-199.994620514454,-1.46991557547311,
4.77667056327245));
#26648=CARTESIAN_POINT('Ctrl Pts',(-199.993854778578,-1.56764391719393,
4.74421450873475));
#26649=CARTESIAN_POINT('Ctrl Pts',(-199.993085898841,-1.66577349952316,
4.71162520025208));
#26650=CARTESIAN_POINT('Ctrl Pts',(-199.992252681875,-1.76292784884562,
4.67603232316609));
#26651=CARTESIAN_POINT('Ctrl Pts',(-199.991362450643,-1.8587399424392,4.63759524240013));
#26652=CARTESIAN_POINT('Ctrl Pts',(-199.991194313101,-1.87683592615673,
4.63033564957001));
#26653=CARTESIAN_POINT('Ctrl Pts',(-199.991024144221,-1.89488408653804,
4.62297473725664));
#26654=CARTESIAN_POINT('Ctrl Pts',(-199.99085199658,-1.91288203555658,4.61551376961371));
#26655=CARTESIAN_POINT('Ctrl Pts',(-199.989904874678,-2.01190315274628,
4.57446501730539));
#26656=CARTESIAN_POINT('Ctrl Pts',(-199.988899457035,-2.10927871154764,
4.53044461549043));
#26657=CARTESIAN_POINT('Ctrl Pts',(-199.987843468119,-2.20502888611135,
4.48349555285956));
#26658=CARTESIAN_POINT('Ctrl Pts',(-199.986757493131,-2.30349800160627,
4.43521331534257));
#26659=CARTESIAN_POINT('Ctrl Pts',(-199.985618017165,-2.40024873744451,
4.38383369995907));
#26660=CARTESIAN_POINT('Ctrl Pts',(-199.984432539851,-2.49528004234097,
4.32935098459506));
#26661=CARTESIAN_POINT('Ctrl Pts',(-199.983247062538,-2.59031134723743,
4.27486826923105));
#26662=CARTESIAN_POINT('Ctrl Pts',(-199.982015562515,-2.68362377968778,
4.21728220597808));
#26663=CARTESIAN_POINT('Ctrl Pts',(-199.980744946282,-2.77518481010207,
4.15653780076889));
#26664=CARTESIAN_POINT('Ctrl Pts',(-199.979687255074,-2.85140239203149,
4.10597271145264));
#26665=CARTESIAN_POINT('Ctrl Pts',(-199.978600516736,-2.9265466732396,4.05311678006709));
#26666=CARTESIAN_POINT('Ctrl Pts',(-199.97749418169,-3.00027821641985,3.99812698221601));
#26667=CARTESIAN_POINT('Ctrl Pts',(-199.976393937536,-3.07360383295553,
3.94343992893212));
#26668=CARTESIAN_POINT('Ctrl Pts',(-199.975274327849,-3.14553183064925,
3.88664264803906));
#26669=CARTESIAN_POINT('Ctrl Pts',(-199.974145117408,-3.21575710395861,
3.8279320050744));
#26670=CARTESIAN_POINT('Ctrl Pts',(-199.973025477985,-3.28538715839498,
3.76971898470472));
#26671=CARTESIAN_POINT('Ctrl Pts',(-199.971896415508,-3.35334289883324,
3.70962515107354));
#26672=CARTESIAN_POINT('Ctrl Pts',(-199.970767675592,-3.41936063468391,
3.64788081857121));
#26673=CARTESIAN_POINT('Ctrl Pts',(-199.970092075881,-3.45887510795394,
3.61092416223028));
#26674=CARTESIAN_POINT('Ctrl Pts',(-199.969416594978,-3.49769595511179,
3.57337692846561));
#26675=CARTESIAN_POINT('Ctrl Pts',(-199.968743327174,-3.53577320409041,
3.53529459150656));
#26676=CARTESIAN_POINT('Ctrl Pts',(-199.968742852571,-3.53580004569161,
3.53526774631872));
#26677=CARTESIAN_POINT('Ctrl Pts',(-199.968742377966,-3.53582688695847,
3.53524090083019));
#26678=CARTESIAN_POINT('Ctrl Pts',(-199.96874190336,-3.53585372789099,3.53521405504099));
#26679=CARTESIAN_POINT('Ctrl Pts',(-199.967444306764,-3.60923812433126,
3.46181638019514));
#26680=CARTESIAN_POINT('Ctrl Pts',(-199.96615206232,-3.68005108080915,3.3861588291228));
#26681=CARTESIAN_POINT('Ctrl Pts',(-199.96487158156,-3.7483671018263,3.30830569199624));
#26682=CARTESIAN_POINT('Ctrl Pts',(-199.963578976183,-3.8173299936106,3.22971537905371));
#26683=CARTESIAN_POINT('Ctrl Pts',(-199.962298340418,-3.88374870870884,
3.14888724765019));
#26684=CARTESIAN_POINT('Ctrl Pts',(-199.961036490355,-3.94766064639338,
3.06585149879162));
#26685=CARTESIAN_POINT('Ctrl Pts',(-199.959767630885,-4.01192760630376,
2.98235449750583));
#26686=CARTESIAN_POINT('Ctrl Pts',(-199.95851774743,-4.07366014499625,2.8966247992817));
#26687=CARTESIAN_POINT('Ctrl Pts',(-199.9572942706,-4.13285266915211,2.80866409485437));
#26688=CARTESIAN_POINT('Ctrl Pts',(-199.957156589108,-4.13951378018764,
2.79876561481302));
#26689=CARTESIAN_POINT('Ctrl Pts',(-199.957019242719,-4.14614267740391,
2.78883885648985));
#26690=CARTESIAN_POINT('Ctrl Pts',(-199.956882242582,-4.1527393159331,2.77888380370217));
#26691=CARTESIAN_POINT('Ctrl Pts',(-199.95544980972,-4.22171181515478,2.6747967194074));
#26692=CARTESIAN_POINT('Ctrl Pts',(-199.954061738656,-4.28685552312269,
2.56806446356432));
#26693=CARTESIAN_POINT('Ctrl Pts',(-199.952733419531,-4.34795058887662,
2.45918047711815));
#26694=CARTESIAN_POINT('Ctrl Pts',(-199.951403408728,-4.40912346210568,
2.350157821731));
#26695=CARTESIAN_POINT('Ctrl Pts',(-199.950133324005,-4.46623711952495,
2.23897859314705));
#26696=CARTESIAN_POINT('Ctrl Pts',(-199.948937830268,-4.51911834064776,
2.12615943202458));
#26697=CARTESIAN_POINT('Ctrl Pts',(-199.948189148319,-4.55223538211244,
2.05550605531406));
#26698=CARTESIAN_POINT('Ctrl Pts',(-199.947469703636,-4.58369344950168,
1.98420989675678));
#26699=CARTESIAN_POINT('Ctrl Pts',(-199.946782884472,-4.61346010601319,
1.91240038831081));
#26700=CARTESIAN_POINT('Ctrl Pts',(-199.945244027512,-4.6801539738286,1.75150714649393));
#26701=CARTESIAN_POINT('Ctrl Pts',(-199.943856293354,-4.7389159061174,1.58668726934914));
#26702=CARTESIAN_POINT('Ctrl Pts',(-199.942652291952,-4.78917780218821,
1.41890182598691));
#26703=CARTESIAN_POINT('Ctrl Pts',(-199.941603884009,-4.83294433847652,
1.27279934538775));
#26704=CARTESIAN_POINT('Ctrl Pts',(-199.940694808944,-4.87026604422707,
1.12444935722674));
#26705=CARTESIAN_POINT('Ctrl Pts',(-199.939946726429,-4.90078596069864,
0.974512902480285));
#26706=CARTESIAN_POINT('Ctrl Pts',(-199.939427256788,-4.92197903733681,
0.870396799172517));
#26707=CARTESIAN_POINT('Ctrl Pts',(-199.938988357527,-4.93977769851255,
0.766104978326001));
#26708=CARTESIAN_POINT('Ctrl Pts',(-199.938631378381,-4.95419932373587,
0.661646608786745));
#26709=CARTESIAN_POINT('Ctrl Pts',(-199.938257638965,-4.96929804824874,
0.552283889931227));
#26710=CARTESIAN_POINT('Ctrl Pts',(-199.937973662438,-4.98069584575212,
0.442738086230268));
#26711=CARTESIAN_POINT('Ctrl Pts',(-199.937782272973,-4.98835300268657,
0.333005356084353));
#26712=CARTESIAN_POINT('Ctrl Pts',(-199.937602385329,-4.99554999187818,
0.229867170516646));
#26713=CARTESIAN_POINT('Ctrl Pts',(-199.937504286432,-4.99944209055195,
0.126563270586194));
#26714=CARTESIAN_POINT('Ctrl Pts',(-199.93749163394,-4.99994428099082,0.023086513920902));
#26715=CARTESIAN_POINT('Ctrl Pts',(-199.937490824953,-4.99997639050698,
0.0164703214711166));
#26716=CARTESIAN_POINT('Ctrl Pts',(-199.937490365772,-4.9999946236966,0.00985342258791087));
#26717=CARTESIAN_POINT('Ctrl Pts',(-199.937490257555,-4.99999895100586,
0.0032358156249388));
#26718=CARTESIAN_POINT('Ctrl Pts',(-199.937490254414,-4.99999907661167,
0.00304373093410148));
#26719=CARTESIAN_POINT('Ctrl Pts',(-199.937490251566,-4.99999919050223,
0.00285164428297918));
#26720=CARTESIAN_POINT('Ctrl Pts',(-199.937490249012,-4.99999929267631,
0.00265955567477993));
#26721=CARTESIAN_POINT('Ctrl Pts',(-199.937489018394,-5.00004851957442,
-0.0898876536395686));
#26722=CARTESIAN_POINT('Ctrl Pts',(-199.937555311217,-4.99741975628316,
-0.182864303586234));
#26723=CARTESIAN_POINT('Ctrl Pts',(-199.937688351934,-4.99210548149748,
-0.275917348301421));
#26724=CARTESIAN_POINT('Ctrl Pts',(-199.93782217992,-4.98675975948198,-0.369521034562259));
#26725=CARTESIAN_POINT('Ctrl Pts',(-199.93802353579,-4.97869670341907,-0.463201601617108));
#26726=CARTESIAN_POINT('Ctrl Pts',(-199.938290146692,-4.96796164028995,
-0.55659875106629));
#26727=CARTESIAN_POINT('Ctrl Pts',(-199.938559009798,-4.95713589231543,
-0.650784876412101));
#26728=CARTESIAN_POINT('Ctrl Pts',(-199.938894221274,-4.94359288496629,
-0.744682325979206));
#26729=CARTESIAN_POINT('Ctrl Pts',(-199.939292143059,-4.92743182600384,
-0.83792723245062));
#26730=CARTESIAN_POINT('Ctrl Pts',(-199.939485856053,-4.91956443285371,
-0.883319947133576));
#26731=CARTESIAN_POINT('Ctrl Pts',(-199.939694412189,-4.91107738229964,
-0.92855814571286));
#26732=CARTESIAN_POINT('Ctrl Pts',(-199.939917296751,-4.90198647167366,
-0.973600817409316));
#26733=CARTESIAN_POINT('Ctrl Pts',(-199.940432998255,-4.88095228142656,
-1.07781877363846));
#26734=CARTESIAN_POINT('Ctrl Pts',(-199.941025461063,-4.8566757112893,-1.18106633068164));
#26735=CARTESIAN_POINT('Ctrl Pts',(-199.941688795583,-4.82922287470041,
-1.28335964233559));
#26736=CARTESIAN_POINT('Ctrl Pts',(-199.94237779903,-4.80070770107679,-1.38961137821365));
#26737=CARTESIAN_POINT('Ctrl Pts',(-199.943143277804,-4.76876581555304,
-1.49483421609362));
#26738=CARTESIAN_POINT('Ctrl Pts',(-199.943979937156,-4.73341334146045,
-1.59903492795587));
#26739=CARTESIAN_POINT('Ctrl Pts',(-199.944816596509,-4.69806086736786,
-1.70323563981812));
#26740=CARTESIAN_POINT('Ctrl Pts',(-199.94572445736,-4.65929760500322,-1.80641482608029));
#26741=CARTESIAN_POINT('Ctrl Pts',(-199.946699239106,-4.6170838617425,-1.90855889410973));
#26742=CARTESIAN_POINT('Ctrl Pts',(-199.947580381328,-4.57892525687886,
-2.00089079434012));
#26743=CARTESIAN_POINT('Ctrl Pts',(-199.948516093726,-4.53794998774401,
-2.09234828148755));
#26744=CARTESIAN_POINT('Ctrl Pts',(-199.949497749995,-4.49428712792918,
-2.18256058586003));
#26745=CARTESIAN_POINT('Ctrl Pts',(-199.950476582457,-4.45074986757737,
-2.27251338783079));
#26746=CARTESIAN_POINT('Ctrl Pts',(-199.951501077833,-4.40454064626135,
-2.36122770153106));
#26747=CARTESIAN_POINT('Ctrl Pts',(-199.952561949386,-4.35583435842811,
-2.44835766799837));
#26748=CARTESIAN_POINT('Ctrl Pts',(-199.953616658333,-4.30741100559012,
-2.53498149618775));
#26749=CARTESIAN_POINT('Ctrl Pts',(-199.954707305064,-4.25651974942602,
-2.62003892222701));
#26750=CARTESIAN_POINT('Ctrl Pts',(-199.955824291176,-4.20337568799156,
-2.70321804011165));
#26751=CARTESIAN_POINT('Ctrl Pts',(-199.956150084159,-4.18787508138827,
-2.72747901582816));
#26752=CARTESIAN_POINT('Ctrl Pts',(-199.95647811572,-4.17218309254555,-2.7515804034736));
#26753=CARTESIAN_POINT('Ctrl Pts',(-199.956808143247,-4.15630571118181,
-2.77551499024965));
#26754=CARTESIAN_POINT('Ctrl Pts',(-199.958041623657,-4.09696387666182,
-2.86497069174285));
#26755=CARTESIAN_POINT('Ctrl Pts',(-199.959307171522,-4.03482709411232,
-2.95241426284234));
#26756=CARTESIAN_POINT('Ctrl Pts',(-199.960597054839,-3.96986498978254,
-3.03782589471581));
#26757=CARTESIAN_POINT('Ctrl Pts',(-199.961908169113,-3.90383363553538,
-3.12464336744474));
#26758=CARTESIAN_POINT('Ctrl Pts',(-199.963244443954,-3.83488312171559,
-3.2093620691339));
#26759=CARTESIAN_POINT('Ctrl Pts',(-199.964598170151,-3.76293631073179,
-3.29192868461025));
#26760=CARTESIAN_POINT('Ctrl Pts',(-199.965951896348,-3.69098949974798,
-3.3744953000866));
#26761=CARTESIAN_POINT('Ctrl Pts',(-199.967323092875,-3.61604622668702,
-3.4549103913015));
#26762=CARTESIAN_POINT('Ctrl Pts',(-199.968704181972,-3.53798640232844,
-3.53307970260756));
#26763=CARTESIAN_POINT('Ctrl Pts',(-199.968708043157,-3.53776816630022,
-3.5332982447343));
#26764=CARTESIAN_POINT('Ctrl Pts',(-199.9687119045,-3.53754990939351,-3.5335167657643));
#26765=CARTESIAN_POINT('Ctrl Pts',(-199.968715766001,-3.53733163160961,
-3.53373526569466));
#26766=CARTESIAN_POINT('Ctrl Pts',(-199.970460080778,-3.43873134294032,
-3.63243590220857));
#26767=CARTESIAN_POINT('Ctrl Pts',(-199.972198400985,-3.33629856007218,
-3.72641353533234));
#26768=CARTESIAN_POINT('Ctrl Pts',(-199.973909045,-3.23039261393604,-3.81566236806452));
#26769=CARTESIAN_POINT('Ctrl Pts',(-199.975658208745,-3.12210191187783,
-3.90692087721395));
#26770=CARTESIAN_POINT('Ctrl Pts',(-199.977378457628,-3.01017939050342,
-3.99323556564552));
#26771=CARTESIAN_POINT('Ctrl Pts',(-199.979046584187,-2.89497003626135,
-4.07456264639649));
#26772=CARTESIAN_POINT('Ctrl Pts',(-199.979597895336,-2.85689366779627,
-4.10144101849774));
#26773=CARTESIAN_POINT('Ctrl Pts',(-199.980143511582,-2.81845800392829,
-4.12777428048652));
#26774=CARTESIAN_POINT('Ctrl Pts',(-199.980682588089,-2.77967472951125,
-4.15355987795727));
#26775=CARTESIAN_POINT('Ctrl Pts',(-199.981936089878,-2.68949290329997,
-4.21351851489069));
#26776=CARTESIAN_POINT('Ctrl Pts',(-199.983159605109,-2.59702475552414,
-4.27078090281776));
#26777=CARTESIAN_POINT('Ctrl Pts',(-199.98434087393,-2.50260165939654,-4.32510605814017));
#26778=CARTESIAN_POINT('Ctrl Pts',(-199.985531674863,-2.40741662703508,
-4.37986958400906));
#26779=CARTESIAN_POINT('Ctrl Pts',(-199.986679525956,-2.31024540313252,
-4.43164800465818));
#26780=CARTESIAN_POINT('Ctrl Pts',(-199.987772232793,-2.2114590901831,-4.48023721382498));
#26781=CARTESIAN_POINT('Ctrl Pts',(-199.988854707903,-2.11359777799008,
-4.52837145049721));
#26782=CARTESIAN_POINT('Ctrl Pts',(-199.989883049618,-2.01415200967174,
-4.57337579852419));
#26783=CARTESIAN_POINT('Ctrl Pts',(-199.990846026127,-1.91350614160602,
-4.61509643178297));
#26784=CARTESIAN_POINT('Ctrl Pts',(-199.991792578594,-1.81457683872722,
-4.65610549895359));
#26785=CARTESIAN_POINT('Ctrl Pts',(-199.992673774464,-1.71473372927819,
-4.69384912860981));
#26786=CARTESIAN_POINT('Ctrl Pts',(-199.993486393832,-1.61399492659733,
-4.72837579234345));
#26787=CARTESIAN_POINT('Ctrl Pts',(-199.994324637517,-1.51007952847902,
-4.7639911849439));
#26788=CARTESIAN_POINT('Ctrl Pts',(-199.99508993585,-1.40521060200091,-4.79618398139478));
#26789=CARTESIAN_POINT('Ctrl Pts',(-199.995777839267,-1.29938616024233,
-4.82495380141363));
#26790=CARTESIAN_POINT('Ctrl Pts',(-199.996465742685,-1.19356171848376,
-4.85372362143249));
#26791=CARTESIAN_POINT('Ctrl Pts',(-199.997076272279,-1.08678118100251,
-4.87907068709403));
#26792=CARTESIAN_POINT('Ctrl Pts',(-199.997603740834,-0.979029072192739,
-4.90093718328894));
#26793=CARTESIAN_POINT('Ctrl Pts',(-199.998041002663,-0.889704535842363,
-4.91906411050914));
#26794=CARTESIAN_POINT('Ctrl Pts',(-199.998421910603,-0.799504709890456,
-4.93483341825751));
#26795=CARTESIAN_POINT('Ctrl Pts',(-199.998743013132,-0.708780351873667,
-4.94811277000276));
#26796=CARTESIAN_POINT('Ctrl Pts',(-199.999062276332,-0.618575678176499,
-4.96131605539684));
#26797=CARTESIAN_POINT('Ctrl Pts',(-199.999322402602,-0.527852889778465,
-4.97205769319153));
#26798=CARTESIAN_POINT('Ctrl Pts',(-199.999521129845,-0.436966717214281,
-4.98025786977575));
#26799=CARTESIAN_POINT('Ctrl Pts',(-199.999718104531,-0.346882062129988,
-4.98838572969523));
#26800=CARTESIAN_POINT('Ctrl Pts',(-199.999854746094,-0.256637304488128,
-4.99401669745692));
#26801=CARTESIAN_POINT('Ctrl Pts',(-199.999930165345,-0.166581446325115,
-4.99712397975926));
#26802=CARTESIAN_POINT('Ctrl Pts',(-199.99997625447,-0.111547809076515,
-4.99902285730641));
#26803=CARTESIAN_POINT('Ctrl Pts',(-199.999999506613,-0.056584759504595,
-4.99998026449961));
#26804=CARTESIAN_POINT('Ctrl Pts',(-199.999999992153,-0.00177162224212468,
-4.99999968613545));
#26805=CARTESIAN_POINT('',(198.037532067764,27.948808427362,-7.5));
#26806=CARTESIAN_POINT('Origin',(6.93889390390723E-15,1.21430643318376E-14,
-7.5));
#26807=CARTESIAN_POINT('',(198.037532067764,27.948808427362,7.5));
#26808=CARTESIAN_POINT('Origin',(6.93889390390723E-15,1.21430643318376E-14,
7.5));
#26809=CARTESIAN_POINT('',(198.037532067764,27.948808427362,-7.5));
#26810=CARTESIAN_POINT('',(-185.006620848663,75.9773008349145,7.5));
#26811=CARTESIAN_POINT('',(-185.006620848663,75.9773008349145,-7.5));
#26812=CARTESIAN_POINT('',(-185.006620848663,75.9773008349145,12.5));
#26813=CARTESIAN_POINT('Origin',(6.93889390390723E-15,1.21430643318376E-14,
-7.5));
#26814=CARTESIAN_POINT('Origin',(6.93889390390723E-15,1.21430643318376E-14,
7.5));
#26815=CARTESIAN_POINT('',(-185.006620848663,-75.9773008349146,-7.5));
#26816=CARTESIAN_POINT('Origin',(6.93889390390723E-15,1.21430643318376E-14,
-7.5));
#26817=CARTESIAN_POINT('',(-185.006620848663,-75.9773008349146,7.5));
#26818=CARTESIAN_POINT('',(-185.006620848663,-75.9773008349146,12.5));
#26819=CARTESIAN_POINT('Origin',(6.93889390390723E-15,1.21430643318376E-14,
7.5));
#26820=CARTESIAN_POINT('',(198.037532067764,-27.948808427362,-7.5));
#26821=CARTESIAN_POINT('Origin',(6.93889390390723E-15,1.21430643318376E-14,
-7.5));
#26822=CARTESIAN_POINT('',(198.037532067764,-27.9488084273619,7.5));
#26823=CARTESIAN_POINT('',(198.037532067764,-27.9488084273619,-7.5));
#26824=CARTESIAN_POINT('Origin',(6.93889390390723E-15,1.21430643318376E-14,
7.5));
#26825=CARTESIAN_POINT('Origin',(0.,0.,7.5));
#26826=CARTESIAN_POINT('',(-181.394623471171,-63.9195500642836,7.5));
#26827=CARTESIAN_POINT('Origin',(-175.75628980623,-72.1784357931688,7.5));
#26828=CARTESIAN_POINT('',(-43.7076833558927,-63.9537123387768,7.5));
#26829=CARTESIAN_POINT('Origin',(-112.576160096458,-164.723060254401,7.5));
#26830=CARTESIAN_POINT('',(43.7076833558926,-63.9537123387769,7.5));
#26831=CARTESIAN_POINT('Origin',(0.,0.,7.5));
#26832=CARTESIAN_POINT('Origin',(112.576160096458,-164.723060254401,7.5));
#26833=CARTESIAN_POINT('Origin',(198.037532067764,4.85052059515657E-14,
7.5));
#26834=CARTESIAN_POINT('',(43.7076833558927,63.9537123387769,7.5));
#26835=CARTESIAN_POINT('Origin',(112.576160096458,164.723060254401,7.5));
#26836=CARTESIAN_POINT('',(-43.7076833558927,63.9537123387769,7.5));
#26837=CARTESIAN_POINT('Origin',(0.,0.,7.5));
#26838=CARTESIAN_POINT('',(-181.394623471171,63.9195500642836,7.5));
#26839=CARTESIAN_POINT('Origin',(-112.576160096458,164.723060254401,7.5));
#26840=CARTESIAN_POINT('Origin',(-175.75628980623,72.1784357931688,7.5));
#26841=CARTESIAN_POINT('',(49.8000928868158,55.4601300422384,7.5));
#26842=CARTESIAN_POINT('',(45.9698706712208,58.6740680906711,7.5));
#26843=CARTESIAN_POINT('',(49.8000928868158,55.4601300422384,7.5));
#26844=CARTESIAN_POINT('',(18.2451455071118,17.854408138354,7.5));
#26845=CARTESIAN_POINT('',(49.8000928868158,55.4601300422384,7.5));
#26846=CARTESIAN_POINT('',(24.7730106681704,6.90671670389171,7.5));
#26847=CARTESIAN_POINT('Origin',(0.745999527119512,1.21430643318376E-14,
7.5));
#26848=CARTESIAN_POINT('',(72.9299279571745,15.3980805296896,7.5));
#26849=CARTESIAN_POINT('',(72.9299279571745,15.3980805296896,7.5));
#26850=CARTESIAN_POINT('',(73.7981688455092,10.4740417646285,7.5));
#26851=CARTESIAN_POINT('',(73.7981688455092,10.4740417646286,7.5));
#26852=CARTESIAN_POINT('',(73.7981688455092,10.4740417646286,7.5));
#26853=CARTESIAN_POINT('',(65.7652614261009,-35.0828400417365,7.5));
#26854=CARTESIAN_POINT('',(65.7652614261009,-35.0828400417365,7.5));
#26855=CARTESIAN_POINT('',(63.265261426101,-39.4129670606588,7.5));
#26856=CARTESIAN_POINT('',(63.2652614261009,-39.4129670606588,7.5));
#26857=CARTESIAN_POINT('',(20.8166938897999,-14.9052751668619,7.5));
#26858=CARTESIAN_POINT('',(63.2652614261009,-39.4129670606588,7.5));
#26859=CARTESIAN_POINT('',(10.9648337349804,-22.8161220945246,7.5));
#26860=CARTESIAN_POINT('Origin',(0.745999527119512,1.21430643318376E-14,
7.5));
#26861=CARTESIAN_POINT('',(27.8282981742883,-69.1481098552981,7.5));
#26862=CARTESIAN_POINT('',(27.8282981742883,-69.1481098552981,7.5));
#26863=CARTESIAN_POINT('',(23.1298350703588,-70.8582105719264,7.5));
#26864=CARTESIAN_POINT('',(23.1298350703588,-70.8582105719264,7.5));
#26865=CARTESIAN_POINT('',(6.21815778991956,-24.393759118817,7.5));
#26866=CARTESIAN_POINT('',(23.1298350703588,-70.8582105719264,7.5));
#26867=CARTESIAN_POINT('',(-6.09183989625028,-24.0467035582886,7.5));
#26868=CARTESIAN_POINT('Origin',(0.745999527119512,1.21430643318376E-14,
7.5));
#26869=CARTESIAN_POINT('',(-23.1298350703578,-70.8582105719268,7.5));
#26870=CARTESIAN_POINT('',(-23.1298350703578,-70.8582105719268,7.5));
#26871=CARTESIAN_POINT('',(-27.8282981742874,-69.1481098552985,7.5));
#26872=CARTESIAN_POINT('',(-27.8282981742874,-69.1481098552985,7.5));
#26873=CARTESIAN_POINT('',(-10.7420901590486,-22.2041391493244,7.5));
#26874=CARTESIAN_POINT('',(-27.8282981742874,-69.1481098552985,7.5));
#26875=CARTESIAN_POINT('',(-19.7626328986541,-14.296712769882,7.5));
#26876=CARTESIAN_POINT('Origin',(0.745999527119512,1.21430643318376E-14,
7.5));
#26877=CARTESIAN_POINT('',(-63.2652614261004,-39.4129670606597,7.5));
#26878=CARTESIAN_POINT('',(-63.2652614261004,-39.4129670606597,7.5));
#26879=CARTESIAN_POINT('',(-65.7652614261004,-35.0828400417375,7.5));
#26880=CARTESIAN_POINT('',(-65.7652614261004,-35.0828400417375,7.5));
#26881=CARTESIAN_POINT('',(-22.2199439289764,-9.94193926282494,7.5));
#26882=CARTESIAN_POINT('',(-65.7652614261004,-35.0828400417375,7.5));
#26883=CARTESIAN_POINT('',(-22.1041836607387,-10.1424419289105,7.5));
#26884=CARTESIAN_POINT('',(-22.2199439289764,-9.94193926282494,7.5));
#26885=CARTESIAN_POINT('',(-24.1016880072274,2.75543539126987,7.50000000000001));
#26886=CARTESIAN_POINT('Origin',(0.745999527119512,1.21430643318376E-14,
7.5));
#26887=CARTESIAN_POINT('',(-24.2802608359423,1.74269855430126,7.5));
#26888=CARTESIAN_POINT('',(-23.4120199476077,6.6667373193623,7.5));
#26889=CARTESIAN_POINT('',(-73.7981688455094,10.4740417646276,7.5));
#26890=CARTESIAN_POINT('',(-73.7981688455094,10.4740417646276,7.5));
#26891=CARTESIAN_POINT('',(-72.9299279571747,15.3980805296886,7.5));
#26892=CARTESIAN_POINT('',(-72.9299279571747,15.3980805296886,7.5));
#26893=CARTESIAN_POINT('',(-23.4120199476077,6.6667373193623,7.5));
#26894=CARTESIAN_POINT('',(-72.9299279571747,15.3980805296886,7.5));
#26895=CARTESIAN_POINT('',(-23.545603499947,5.90914734758,7.50000000000001));
#26896=CARTESIAN_POINT('',(-23.4120199476077,6.6667373193623,7.5));
#26897=CARTESIAN_POINT('',(-17.5548310250611,17.0317233743498,7.5));
#26898=CARTESIAN_POINT('Origin',(0.745999527119512,1.21430643318376E-14,
7.5));
#26899=CARTESIAN_POINT('',(-49.8000928868165,55.4601300422377,7.5));
#26900=CARTESIAN_POINT('',(-49.8000928868165,55.4601300422377,7.5));
#26901=CARTESIAN_POINT('',(-45.9698706712216,58.6740680906704,7.5));
#26902=CARTESIAN_POINT('',(-45.9698706712216,58.6740680906704,7.5));
#26903=CARTESIAN_POINT('',(-13.7984652228223,20.3336800687357,7.5));
#26904=CARTESIAN_POINT('',(-45.9698706712216,58.6740680906704,7.5));
#26905=CARTESIAN_POINT('',(-2.5,24.7883740303785,7.5));
#26906=CARTESIAN_POINT('Origin',(0.745999527119512,1.21430643318376E-14,
7.5));
#26907=CARTESIAN_POINT('',(-2.5,74.4958071023965,7.5));
#26908=CARTESIAN_POINT('',(-2.5,74.4958071023965,7.5));
#26909=CARTESIAN_POINT('',(2.5,74.4958071023965,7.5));
#26910=CARTESIAN_POINT('',(2.5,74.4958071023965,7.5));
#26911=CARTESIAN_POINT('',(2.5,24.9383937401978,7.5));
#26912=CARTESIAN_POINT('',(2.5,74.4958071023965,7.5));
#26913=CARTESIAN_POINT('',(14.3410668781608,20.9803275408334,7.5));
#26914=CARTESIAN_POINT('Origin',(0.745999527119512,1.21430643318376E-14,
7.5));
#26915=CARTESIAN_POINT('',(45.9698706712208,58.6740680906711,7.5));
#26916=CARTESIAN_POINT('Origin',(0.745999527119512,1.21430643318376E-14,
-78.2106781186548));
#26917=CARTESIAN_POINT('',(18.2451455071118,17.854408138354,15.));
#26918=CARTESIAN_POINT('',(18.2451455071118,17.854408138354,-78.2106781186548));
#26919=CARTESIAN_POINT('',(24.7730106681704,6.90671670389171,15.));
#26920=CARTESIAN_POINT('Origin',(0.745999527119512,1.21430643318376E-14,
15.));
#26921=CARTESIAN_POINT('',(24.7730106681704,6.90671670389171,-78.2106781186548));
#26922=CARTESIAN_POINT('Origin',(0.745999527119512,1.21430643318376E-14,
-78.2106781186548));
#26923=CARTESIAN_POINT('',(20.8166938897999,-14.9052751668619,15.));
#26924=CARTESIAN_POINT('',(20.8166938897999,-14.9052751668619,-78.2106781186548));
#26925=CARTESIAN_POINT('',(10.9648337349804,-22.8161220945246,15.));
#26926=CARTESIAN_POINT('Origin',(0.745999527119512,1.21430643318376E-14,
15.));
#26927=CARTESIAN_POINT('',(10.9648337349804,-22.8161220945246,-78.2106781186548));
#26928=CARTESIAN_POINT('Origin',(0.745999527119512,1.21430643318376E-14,
-78.2106781186548));
#26929=CARTESIAN_POINT('',(6.21815778991956,-24.393759118817,15.));
#26930=CARTESIAN_POINT('',(6.21815778991956,-24.393759118817,-78.2106781186548));
#26931=CARTESIAN_POINT('',(-6.09183989625028,-24.0467035582886,15.));
#26932=CARTESIAN_POINT('Origin',(0.745999527119512,1.21430643318376E-14,
15.));
#26933=CARTESIAN_POINT('',(-6.09183989625028,-24.0467035582886,-78.2106781186548));
#26934=CARTESIAN_POINT('Origin',(0.745999527119512,1.21430643318376E-14,
-78.2106781186548));
#26935=CARTESIAN_POINT('',(-10.7420901590486,-22.2041391493244,15.));
#26936=CARTESIAN_POINT('',(-10.7420901590486,-22.2041391493244,-78.2106781186548));
#26937=CARTESIAN_POINT('',(-19.7626328986541,-14.296712769882,15.));
#26938=CARTESIAN_POINT('Origin',(0.745999527119512,1.21430643318376E-14,
15.));
#26939=CARTESIAN_POINT('',(-19.7626328986541,-14.296712769882,-78.2106781186548));
#26940=CARTESIAN_POINT('Origin',(0.745999527119512,1.21430643318376E-14,
-78.2106781186548));
#26941=CARTESIAN_POINT('',(-22.1041836607387,-10.1424419289105,15.));
#26942=CARTESIAN_POINT('',(-22.1041836607387,-10.1424419289104,-78.2106781186548));
#26943=CARTESIAN_POINT('',(-24.1016880072274,2.75543539126994,15.));
#26944=CARTESIAN_POINT('Origin',(0.745999527119512,1.21430643318376E-14,
15.));
#26945=CARTESIAN_POINT('',(-24.1016880072274,2.75543539126993,-78.2106781186548));
#26946=CARTESIAN_POINT('Origin',(0.745999527119512,1.21430643318376E-14,
-78.2106781186548));
#26947=CARTESIAN_POINT('',(14.3410668781608,20.9803275408334,15.));
#26948=CARTESIAN_POINT('',(14.3410668781608,20.9803275408334,-78.2106781186548));
#26949=CARTESIAN_POINT('',(2.5,24.9383937401978,15.));
#26950=CARTESIAN_POINT('',(2.5,24.9383937401978,-78.2106781186548));
#26951=CARTESIAN_POINT('Origin',(0.745999527119512,1.21430643318376E-14,
15.));
#26952=CARTESIAN_POINT('Origin',(0.745999527119512,1.21430643318376E-14,
-78.2106781186548));
#26953=CARTESIAN_POINT('',(-23.545603499947,5.90914734757994,15.));
#26954=CARTESIAN_POINT('',(-23.545603499947,5.90914734757994,-78.2106781186548));
#26955=CARTESIAN_POINT('',(-17.5548310250611,17.0317233743498,15.));
#26956=CARTESIAN_POINT('Origin',(0.745999527119512,1.21430643318376E-14,
15.));
#26957=CARTESIAN_POINT('',(-17.5548310250611,17.0317233743498,-78.2106781186548));
#26958=CARTESIAN_POINT('Origin',(0.745999527119512,1.21430643318376E-14,
-78.2106781186548));
#26959=CARTESIAN_POINT('',(-13.7984652228223,20.3336800687357,15.));
#26960=CARTESIAN_POINT('',(-13.7984652228223,20.3336800687357,-78.2106781186548));
#26961=CARTESIAN_POINT('',(-2.5,24.7883740303784,15.));
#26962=CARTESIAN_POINT('Origin',(0.745999527119512,1.21430643318376E-14,
15.));
#26963=CARTESIAN_POINT('',(-2.5,24.7883740303784,-78.2106781186548));
#26964=CARTESIAN_POINT('Origin',(0.,0.,12.5));
#26965=CARTESIAN_POINT('Origin',(0.,0.,-12.5));
#26966=CARTESIAN_POINT('Origin',(-112.576160096458,-164.723060254401,7.5));
#26967=CARTESIAN_POINT('',(-181.394623471171,-63.9195500642836,-7.5));
#26968=CARTESIAN_POINT('',(-181.394623471171,-63.9195500642835,7.5));
#26969=CARTESIAN_POINT('',(-43.7076833558927,-63.9537123387768,-7.5));
#26970=CARTESIAN_POINT('Origin',(-112.576160096458,-164.723060254401,-7.5));
#26971=CARTESIAN_POINT('',(-43.7076833558927,-63.9537123387768,7.5));
#26972=CARTESIAN_POINT('Origin',(0.,0.,7.5));
#26973=CARTESIAN_POINT('',(43.7076833558926,-63.9537123387769,-7.5));
#26974=CARTESIAN_POINT('Origin',(0.,0.,-7.5));
#26975=CARTESIAN_POINT('',(43.7076833558926,-63.9537123387769,7.5));
#26976=CARTESIAN_POINT('Origin',(112.576160096458,-164.723060254401,7.5));
#26977=CARTESIAN_POINT('Origin',(112.576160096458,-164.723060254401,-7.5));
#26978=CARTESIAN_POINT('Origin',(112.576160096458,164.723060254401,7.5));
#26979=CARTESIAN_POINT('',(43.7076833558927,63.9537123387769,-7.5));
#26980=CARTESIAN_POINT('Origin',(112.576160096458,164.723060254401,-7.5));
#26981=CARTESIAN_POINT('',(43.7076833558927,63.9537123387769,7.5));
#26982=CARTESIAN_POINT('Origin',(0.,0.,7.5));
#26983=CARTESIAN_POINT('',(-43.7076833558927,63.9537123387769,-7.5));
#26984=CARTESIAN_POINT('Origin',(0.,0.,-7.5));
#26985=CARTESIAN_POINT('',(-43.7076833558927,63.9537123387769,7.5));
#26986=CARTESIAN_POINT('Origin',(-112.576160096458,164.723060254401,7.5));
#26987=CARTESIAN_POINT('',(-181.394623471171,63.9195500642836,-7.5));
#26988=CARTESIAN_POINT('Origin',(-112.576160096458,164.723060254401,-7.5));
#26989=CARTESIAN_POINT('',(-181.394623471171,63.9195500642836,7.5));
#26990=CARTESIAN_POINT('Origin',(0.,0.,-7.5));
#26991=CARTESIAN_POINT('Origin',(-175.75628980623,72.1784357931688,-7.5));
#26992=CARTESIAN_POINT('Origin',(198.037532067764,4.85052059515657E-14,
-7.5));
#26993=CARTESIAN_POINT('Origin',(-175.75628980623,-72.1784357931688,-7.5));
#26994=CARTESIAN_POINT('',(2.47860448411075,21.6999127067652,-7.5));
#26995=CARTESIAN_POINT('',(2.47860448411075,0.,-7.5));
#26996=CARTESIAN_POINT('',(-2.0402937480676,21.6999127067652,-7.5));
#26997=CARTESIAN_POINT('',(0.,21.6999127067652,-7.5));
#26998=CARTESIAN_POINT('',(-2.0402937480676,0.,-7.5));
#26999=CARTESIAN_POINT('Origin',(0.,0.,15.));
#27000=CARTESIAN_POINT('',(18.4844395432205,18.139587665573,15.));
#27001=CARTESIAN_POINT('',(17.4795738527292,16.9420353688553,15.));
#27002=CARTESIAN_POINT('',(14.6542173276256,21.3535257140057,15.));
#27003=CARTESIAN_POINT('',(18.4844395432205,18.139587665573,15.));
#27004=CARTESIAN_POINT('',(13.6493516371343,20.1559734172879,15.));
#27005=CARTESIAN_POINT('',(2.5,25.7772990420638,15.));
#27006=CARTESIAN_POINT('',(2.5,24.2140055445719,15.));
#27007=CARTESIAN_POINT('',(-2.5,25.7772990420638,15.));
#27008=CARTESIAN_POINT('',(2.5,25.7772990420638,15.));
#27009=CARTESIAN_POINT('',(-2.5,24.2140055445719,15.));
#27010=CARTESIAN_POINT('',(-14.6542173276259,21.3535257140055,15.));
#27011=CARTESIAN_POINT('',(-13.6493516371345,20.1559734172877,15.));
#27012=CARTESIAN_POINT('',(-18.4844395432208,18.1395876655728,15.));
#27013=CARTESIAN_POINT('',(-14.6542173276259,21.3535257140055,15.));
#27014=CARTESIAN_POINT('',(-17.4795738527294,16.942035368855,15.));
#27015=CARTESIAN_POINT('',(-23.4120199476077,6.6667373193623,15.));
#27016=CARTESIAN_POINT('',(-23.4120199476077,6.6667373193623,15.));
#27017=CARTESIAN_POINT('',(-24.9515635041713,6.93820038636033,15.));
#27018=CARTESIAN_POINT('',(-23.4120199476077,6.6667373193623,15.));
#27019=CARTESIAN_POINT('',(-25.8198043925059,2.01416162129929,15.));
#27020=CARTESIAN_POINT('',(-24.9515635041713,6.93820038636033,15.));
#27021=CARTESIAN_POINT('',(-24.2802608359423,1.74269855430126,15.));
#27022=CARTESIAN_POINT('',(-24.2802608359423,1.74269855430126,15.));
#27023=CARTESIAN_POINT('',(-23.4120199476077,6.6667373193623,15.));
#27024=CARTESIAN_POINT('',(-22.2199439289764,-9.94193926282494,15.));
#27025=CARTESIAN_POINT('',(-22.2199439289764,-9.94193926282494,15.));
#27026=CARTESIAN_POINT('',(-23.5737958113755,-10.7235860115709,15.));
#27027=CARTESIAN_POINT('',(-22.2199439289764,-9.94193926282494,15.));
#27028=CARTESIAN_POINT('',(-21.0737958113755,-15.0537130304931,15.));
#27029=CARTESIAN_POINT('',(-23.5737958113755,-10.7235860115709,15.));
#27030=CARTESIAN_POINT('',(-19.7199439289764,-14.2720662817471,15.));
#27031=CARTESIAN_POINT('',(-11.1655870648799,-23.3676873353049,15.));
#27032=CARTESIAN_POINT('',(-10.6309091988076,-21.8986719715891,15.));
#27033=CARTESIAN_POINT('',(-6.46712396095037,-25.0777880519332,15.));
#27034=CARTESIAN_POINT('',(-11.1655870648799,-23.3676873353049,15.));
#27035=CARTESIAN_POINT('',(-5.93244609487809,-23.6087726882175,15.));
#27036=CARTESIAN_POINT('',(6.4671239609507,-25.0777880519331,15.));
#27037=CARTESIAN_POINT('',(5.93244609487841,-23.6087726882174,15.));
#27038=CARTESIAN_POINT('',(11.1655870648802,-23.3676873353048,15.));
#27039=CARTESIAN_POINT('',(6.4671239609507,-25.0777880519331,15.));
#27040=CARTESIAN_POINT('',(10.6309091988079,-21.898671971589,15.));
#27041=CARTESIAN_POINT('',(21.0737958113757,-15.0537130304928,15.));
#27042=CARTESIAN_POINT('',(19.7199439289766,-14.2720662817468,15.));
#27043=CARTESIAN_POINT('',(23.5737958113756,-10.7235860115706,15.));
#27044=CARTESIAN_POINT('',(21.0737958113757,-15.0537130304928,15.));
#27045=CARTESIAN_POINT('',(22.2199439289766,-9.94193926282463,15.));
#27046=CARTESIAN_POINT('',(25.8198043925059,2.01416162129963,15.));
#27047=CARTESIAN_POINT('',(24.2802608359423,1.74269855430158,15.));
#27048=CARTESIAN_POINT('',(24.9515635041712,6.93820038636067,15.));
#27049=CARTESIAN_POINT('',(25.8198043925059,2.01416162129963,15.));
#27050=CARTESIAN_POINT('',(23.4120199476076,6.66673731936261,15.));
#27051=CARTESIAN_POINT('',(2.47860448411075,21.6999127067652,15.));
#27052=CARTESIAN_POINT('',(2.47860448411075,0.,15.));
#27053=CARTESIAN_POINT('',(-2.0402937480676,21.6999127067652,15.));
#27054=CARTESIAN_POINT('',(-2.0402937480676,0.,15.));
#27055=CARTESIAN_POINT('',(0.,21.6999127067652,15.));
#27056=CARTESIAN_POINT('Origin',(198.037532067764,4.85052059515657E-14,
-7.5));
#27057=CARTESIAN_POINT('Origin',(2.5,25.7772990420638,15.));
#27058=CARTESIAN_POINT('',(-2.5,25.7772990420638,15.));
#27059=CARTESIAN_POINT('',(2.5,25.7772990420638,15.));
#27060=CARTESIAN_POINT('Origin',(2.5,0.,0.));
#27061=CARTESIAN_POINT('Origin',(-2.5,0.,0.));
#27062=CARTESIAN_POINT('Origin',(-14.6542173276259,21.3535257140055,15.));
#27063=CARTESIAN_POINT('',(-18.4844395432208,18.1395876655728,15.));
#27064=CARTESIAN_POINT('',(-14.6542173276259,21.3535257140055,15.));
#27065=CARTESIAN_POINT('Origin',(1.91511110779744,1.60696902421635,0.));
#27066=CARTESIAN_POINT('Origin',(-1.91511110779744,-1.60696902421635,0.));
#27067=CARTESIAN_POINT('Origin',(-23.4120199476077,6.6667373193623,7.5));
#27068=CARTESIAN_POINT('',(-24.2802608359423,1.74269855430126,7.5));
#27069=CARTESIAN_POINT('Origin',(-23.4120199476077,6.6667373193623,7.5));
#27070=CARTESIAN_POINT('',(-23.4120199476077,6.6667373193623,7.5));
#27071=CARTESIAN_POINT('Origin',(-24.9515635041713,6.93820038636033,15.));
#27072=CARTESIAN_POINT('',(-25.8198043925059,2.01416162129929,15.));
#27073=CARTESIAN_POINT('',(-24.9515635041713,6.93820038636033,15.));
#27074=CARTESIAN_POINT('Origin',(0.434120444167318,2.46201938253052,0.));
#27075=CARTESIAN_POINT('Origin',(-0.434120444167318,-2.46201938253052,0.));
#27076=CARTESIAN_POINT('Origin',(-22.2199439289764,-9.94193926282494,7.5));
#27077=CARTESIAN_POINT('',(-22.2199439289764,-9.94193926282494,7.5));
#27078=CARTESIAN_POINT('Origin',(-23.5737958113755,-10.7235860115709,15.));
#27079=CARTESIAN_POINT('',(-21.0737958113755,-15.0537130304931,15.));
#27080=CARTESIAN_POINT('',(-23.5737958113755,-10.7235860115709,15.));
#27081=CARTESIAN_POINT('Origin',(-1.25000000000001,2.16506350946109,0.));
#27082=CARTESIAN_POINT('Origin',(1.25000000000001,-2.16506350946109,0.));
#27083=CARTESIAN_POINT('Origin',(-11.1655870648799,-23.3676873353049,15.));
#27084=CARTESIAN_POINT('',(-6.46712396095037,-25.0777880519332,15.));
#27085=CARTESIAN_POINT('',(-11.1655870648799,-23.3676873353049,15.));
#27086=CARTESIAN_POINT('Origin',(-2.34923155196478,0.855050358314158,0.));
#27087=CARTESIAN_POINT('Origin',(2.34923155196478,-0.855050358314158,0.));
#27088=CARTESIAN_POINT('Origin',(6.4671239609507,-25.0777880519331,15.));
#27089=CARTESIAN_POINT('',(11.1655870648802,-23.3676873353048,15.));
#27090=CARTESIAN_POINT('',(6.4671239609507,-25.0777880519331,15.));
#27091=CARTESIAN_POINT('Origin',(-2.34923155196477,-0.855050358314189,0.));
#27092=CARTESIAN_POINT('Origin',(2.34923155196477,0.855050358314189,0.));
#27093=CARTESIAN_POINT('Origin',(21.0737958113757,-15.0537130304928,15.));
#27094=CARTESIAN_POINT('',(23.5737958113756,-10.7235860115706,15.));
#27095=CARTESIAN_POINT('',(21.0737958113757,-15.0537130304928,15.));
#27096=CARTESIAN_POINT('Origin',(-1.24999999999998,-2.16506350946111,0.));
#27097=CARTESIAN_POINT('Origin',(1.24999999999998,2.16506350946111,0.));
#27098=CARTESIAN_POINT('Origin',(25.8198043925059,2.01416162129963,15.));
#27099=CARTESIAN_POINT('',(24.9515635041712,6.93820038636067,15.));
#27100=CARTESIAN_POINT('',(25.8198043925059,2.01416162129963,15.));
#27101=CARTESIAN_POINT('Origin',(0.434120444167351,-2.46201938253052,0.));
#27102=CARTESIAN_POINT('Origin',(-0.434120444167351,2.46201938253052,0.));
#27103=CARTESIAN_POINT('Origin',(18.4844395432205,18.139587665573,15.));
#27104=CARTESIAN_POINT('',(14.6542173276256,21.3535257140057,15.));
#27105=CARTESIAN_POINT('',(18.4844395432205,18.139587665573,15.));
#27106=CARTESIAN_POINT('Origin',(1.91511110779746,-1.60696902421633,0.));
#27107=CARTESIAN_POINT('Origin',(-1.91511110779746,1.60696902421633,0.));
#27108=CARTESIAN_POINT('Ctrl Pts',(203.999999992307,-0.00177162224216467,
-4.99999968613545));
#27109=CARTESIAN_POINT('Ctrl Pts',(199.974620125013,-0.00177162224216467,
-4.99999968613545));
#27110=CARTESIAN_POINT('Ctrl Pts',(204.000011327375,1.30344668978613,-5.00046215692299));
#27111=CARTESIAN_POINT('Ctrl Pts',(199.974631460081,1.30344668978613,-5.00046215692299));
#27112=CARTESIAN_POINT('Ctrl Pts',(203.985401744253,2.60919356973883,-4.46008193194717));
#27113=CARTESIAN_POINT('Ctrl Pts',(199.960021876959,2.60919356973883,-4.46008193194717));
#27114=CARTESIAN_POINT('Ctrl Pts',(203.953438052627,4.45501092726816,-2.61784253956751));
#27115=CARTESIAN_POINT('Ctrl Pts',(199.928058185333,4.45501092726816,-2.61784253956751));
#27116=CARTESIAN_POINT('Ctrl Pts',(203.938749239315,4.99865586979689,-1.32397596744565));
#27117=CARTESIAN_POINT('Ctrl Pts',(199.913369372021,4.99865586979689,-1.32397596744565));
#27118=CARTESIAN_POINT('Ctrl Pts',(203.938683457647,5.00133895697019,1.31380421087806));
#27119=CARTESIAN_POINT('Ctrl Pts',(199.913303590353,5.00133895697019,1.31380421087806));
#27120=CARTESIAN_POINT('Ctrl Pts',(203.953309177856,4.46081412818035,2.60877766178233));
#27121=CARTESIAN_POINT('Ctrl Pts',(199.927929310562,4.46081412818035,2.60877766178233));
#27122=CARTESIAN_POINT('Ctrl Pts',(203.985313878591,2.61589547515511,4.45664385360227));
#27123=CARTESIAN_POINT('Ctrl Pts',(199.959934011297,2.61589547515511,4.45664385360227));
#27124=CARTESIAN_POINT('Ctrl Pts',(204.,1.32135029102454,5.));
#27125=CARTESIAN_POINT('Ctrl Pts',(199.974620132706,1.32135029102454,5.));
#27126=CARTESIAN_POINT('Ctrl Pts',(204.,2.16840434497101E-16,5.));
#27127=CARTESIAN_POINT('Ctrl Pts',(199.974620132706,2.16840434497101E-16,
5.));
#27128=CARTESIAN_POINT('Origin',(-175.75628980623,-72.1784357931688,12.5));
#27129=CARTESIAN_POINT('Origin',(-175.75628980623,72.1784357931688,7.5));
#27130=CARTESIAN_POINT('Ctrl Pts',(-204.,1.12757025938492E-14,5.));
#27131=CARTESIAN_POINT('Ctrl Pts',(-199.97462301248,1.12757025938492E-14,
5.));
#27132=CARTESIAN_POINT('Ctrl Pts',(-204.,-1.32135029102452,5.));
#27133=CARTESIAN_POINT('Ctrl Pts',(-199.97462301248,-1.32135029102452,5.));
#27134=CARTESIAN_POINT('Ctrl Pts',(-203.985345962115,-2.61339289425714,
4.45784180166548));
#27135=CARTESIAN_POINT('Ctrl Pts',(-199.959968974596,-2.61339289425714,
4.45784180166548));
#27136=CARTESIAN_POINT('Ctrl Pts',(-203.95336383834,-4.45831456152484,2.61258630841651));
#27137=CARTESIAN_POINT('Ctrl Pts',(-199.92798685082,-4.45831456152484,2.61258630841651));
#27138=CARTESIAN_POINT('Ctrl Pts',(-203.938733312599,-4.99930548519225,
1.30702665821118));
#27139=CARTESIAN_POINT('Ctrl Pts',(-199.913356325079,-4.99930548519225,
1.30702665821118));
#27140=CARTESIAN_POINT('Ctrl Pts',(-203.938699292213,-5.00069310016037,
-1.30170754686162));
#27141=CARTESIAN_POINT('Ctrl Pts',(-199.913322304693,-5.00069310016037,
-1.30170754686162));
#27142=CARTESIAN_POINT('Ctrl Pts',(-203.953150206633,-4.47024776275285,
-2.59986968375127));
#27143=CARTESIAN_POINT('Ctrl Pts',(-199.927773219114,-4.47024776275285,
-2.59986968375127));
#27144=CARTESIAN_POINT('Ctrl Pts',(-203.985508343536,-2.60441550046637,
-4.46760084763805));
#27145=CARTESIAN_POINT('Ctrl Pts',(-199.960131356017,-2.60441550046637,
-4.46760084763805));
#27146=CARTESIAN_POINT('Ctrl Pts',(-203.99998865724,-1.30698993427041,-4.99953721534794));
#27147=CARTESIAN_POINT('Ctrl Pts',(-199.97461166972,-1.30698993427041,-4.99953721534794));
#27148=CARTESIAN_POINT('Ctrl Pts',(-204.000000269508,0.0301477011414563,
-5.00001099593282));
#27149=CARTESIAN_POINT('Ctrl Pts',(-199.974623281988,0.0301477011414563,
-5.00001099593282));
#27150=CARTESIAN_POINT('Ctrl Pts',(-203.999991802598,0.0620673406376593,
-4.9996988521178));
#27151=CARTESIAN_POINT('Ctrl Pts',(-199.974614815078,0.0620673406376593,
-4.9996988521178));
#27152=CARTESIAN_POINT('Ctrl Pts',(-203.999974785344,0.0939816893050483,
-4.9990655962846));
#27153=CARTESIAN_POINT('Ctrl Pts',(-199.974597797824,0.0939816893050483,
-4.9990655962846));
#27154=CARTESIAN_POINT('Origin',(2.47860448411075,13.6831560121067,-15.));
#27155=CARTESIAN_POINT('',(2.47860448411075,21.6999127067652,-15.));
#27156=CARTESIAN_POINT('Origin',(-2.0402937480676,13.6831560121067,-15.));
#27157=CARTESIAN_POINT('',(-2.0402937480676,21.6999127067652,-15.));
#27158=CARTESIAN_POINT('Origin',(-2.0402937480676,21.6999127067652,-15.));
#39944=UNCERTAINTY_MEASURE_WITH_UNIT(LENGTH_MEASURE(0.01),#39960,
'DISTANCE_ACCURACY_VALUE',
'Maximum model space distance between geometric entities at asserted c
onnectivities');
#39950=UNCERTAINTY_MEASURE_WITH_UNIT(LENGTH_MEASURE(0.01),#39960,
'DISTANCE_ACCURACY_VALUE',
'Maximum model space distance between geometric entities at asserted c
onnectivities');
#39953=(
GEOMETRIC_REPRESENTATION_CONTEXT(3)
GLOBAL_UNCERTAINTY_ASSIGNED_CONTEXT((#39944))
GLOBAL_UNIT_ASSIGNED_CONTEXT((#39960,#39962,#39963))
REPRESENTATION_CONTEXT('','3D')
);
#39959=(
GEOMETRIC_REPRESENTATION_CONTEXT(3)
GLOBAL_UNCERTAINTY_ASSIGNED_CONTEXT((#39950))
GLOBAL_UNIT_ASSIGNED_CONTEXT((#39960,#39962,#39963))
REPRESENTATION_CONTEXT('','3D')
);
#39960=(
LENGTH_UNIT()
NAMED_UNIT(*)
SI_UNIT(.MILLI.,.METRE.)
);
#39962=(
NAMED_UNIT(*)
PLANE_ANGLE_UNIT()
SI_UNIT($,.RADIAN.)
);
#39963=(
NAMED_UNIT(*)
SI_UNIT($,.STERADIAN.)
SOLID_ANGLE_UNIT()
);
#39966=SHAPE_DEFINITION_REPRESENTATION(#39974,#40003);
#39974=PRODUCT_DEFINITION_SHAPE('',$,#40012);
#40003=SHAPE_REPRESENTATION('',(#18536),#39953);
#40009=PRODUCT_DEFINITION_CONTEXT('part definition',#40035,'design');
#40012=PRODUCT_DEFINITION('Central Rotor Drive Shaft',
'Central Rotor Drive Shaft',#40020,#40009);
#40020=PRODUCT_DEFINITION_FORMATION('',$,#40039);
#40035=APPLICATION_CONTEXT(
'Core Data for Automotive Mechanical Design Process');
#40036=PRODUCT_CONTEXT('part definition',#40035,'mechanical');
#40039=PRODUCT('Central Rotor Drive Shaft','Central Rotor Drive Shaft',
$,(#40036));
#40046=PRESENTATION_STYLE_ASSIGNMENT((#40048));
#40048=SURFACE_STYLE_USAGE(.BOTH.,#40050);
#40050=SURFACE_SIDE_STYLE('',(#40052));
#40052=SURFACE_STYLE_FILL_AREA(#40054);
#40054=FILL_AREA_STYLE('Opaque(202,209,238)',(#40056));
#40056=FILL_AREA_STYLE_COLOUR('Opaque(202,209,238)',#40058);
#40058=COLOUR_RGB('Opaque(202,209,238)', 0.66274510, 0.83137255, 0.94901961);
ENDSEC;
END-ISO-10303-21;
